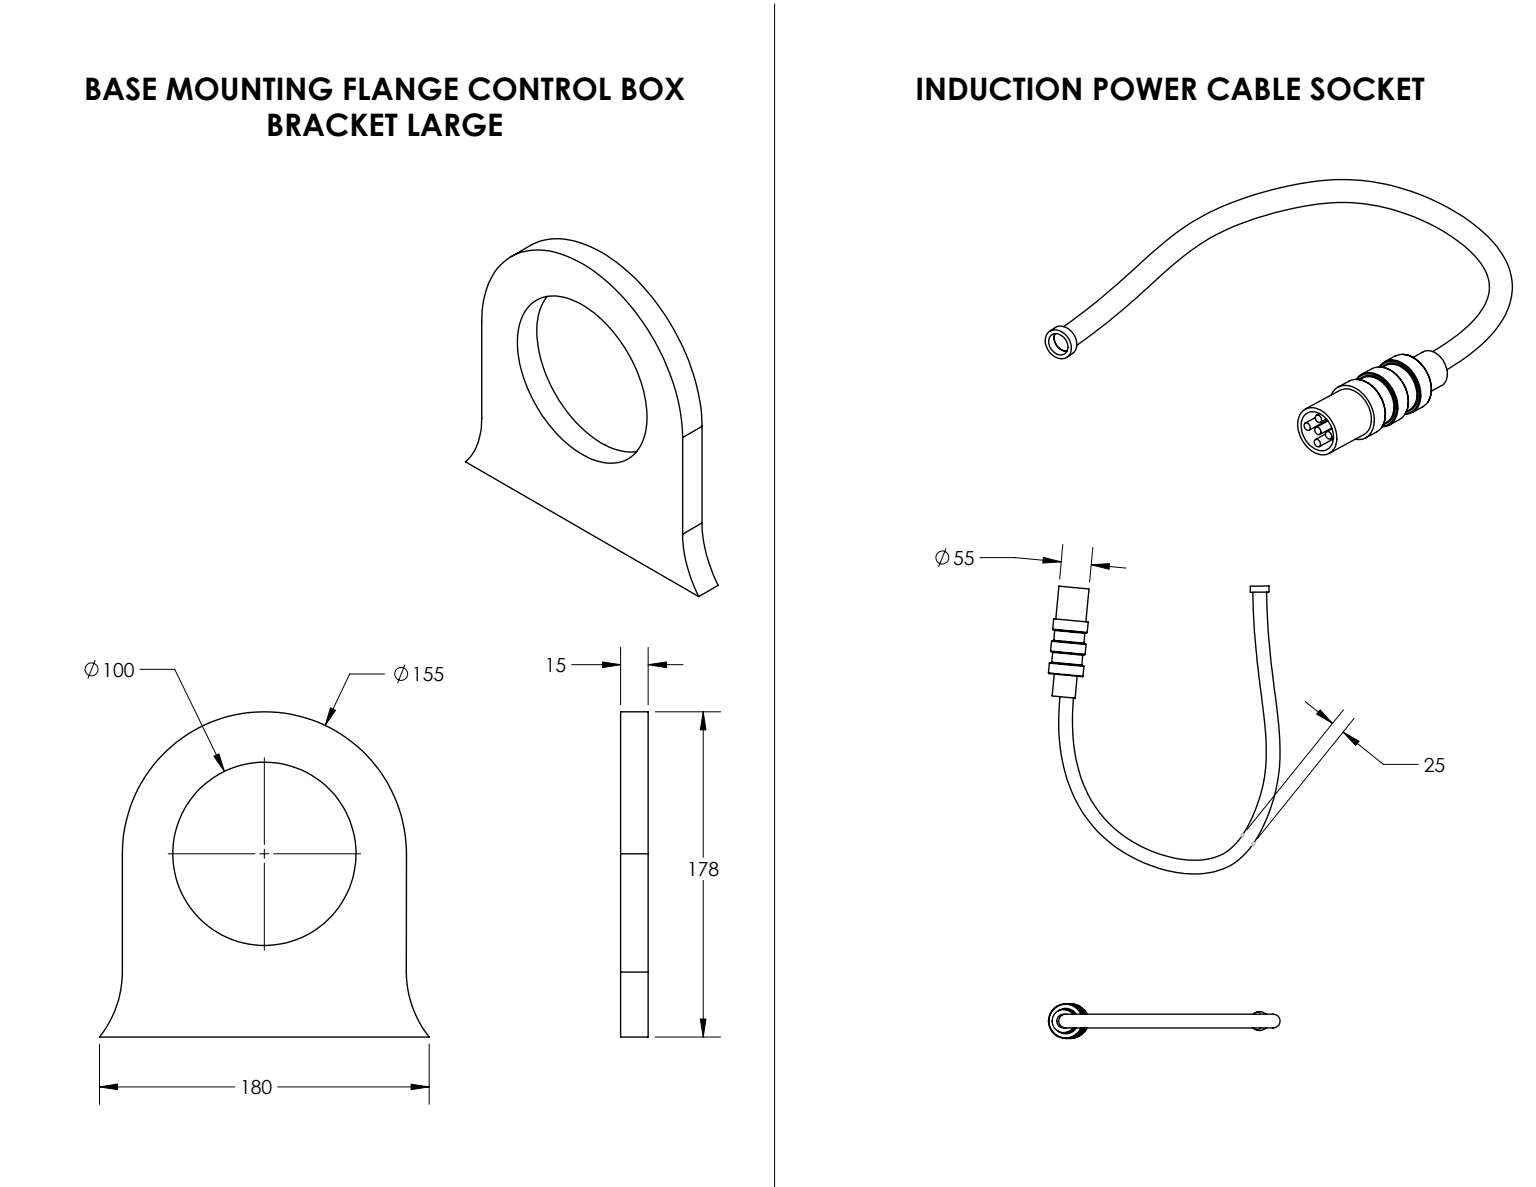
ISO-10303-21;
HEADER;
FILE_DESCRIPTION (('STEP AP214'),
    '1' );
FILE_NAME ('Induction Power Cable Socket.step',
    '2026-10-28T18:30:06',
    ( '' ),
    ( '' ),
    'SwSTEP 2.0',
    'SolidWorks 2024',
    '' );
FILE_SCHEMA (( 'AUTOMOTIVE_DESIGN' ));
ENDSEC;

DATA;
#1=CARTESIAN_POINT ( 'NONE',  ( -382.0077566144223624, 5.421010862429173848E-17, 175.3290427019271078 ) ) ;
#5=DIRECTION ( 'NONE',  ( -0.9955873536034884896, 5.465719896581968711E-31, -0.09383933793885443353 ) ) ;
#8=VERTEX_POINT ( 'NONE', #1404 ) ;
#12=DIRECTION ( 'NONE',  ( -0.09383933793885568253, 2.673190762809473730E-31, 0.9955873536034882676 ) ) ;
#17=CARTESIAN_POINT ( 'NONE',  ( -86.97194166595129161, 3.740497495074990297E-15, 531.0655262460708173 ) ) ;
#18=CARTESIAN_POINT ( 'NONE',  ( -367.0460729392618759, 0.000000000000000000, 268.0688838304710089 ) ) ;
#19=AXIS2_PLACEMENT_3D ( 'NONE', #2675, #4355, #3941 ) ;
#24=CIRCLE ( 'NONE', #2310, 4.382543221487789964 ) ;
#26=ORIENTED_EDGE ( 'NONE', *, *, #5308, .T. ) ;
#30=DIRECTION ( 'NONE',  ( 0.09383933793885537722, -2.626968444144180508E-31, -0.9955873536034883786 ) ) ;
#32=DIRECTION ( 'NONE',  ( 0.09383933793885537722, -2.626968444144180508E-31, -0.9955873536034883786 ) ) ;
#34=CARTESIAN_POINT ( 'NONE',  ( -346.0119820531829191, 0.000000000000000000, 118.4559012928527721 ) ) ;
#35=CIRCLE ( 'NONE', #3119, 30.50000000000124345 ) ;
#36=AXIS2_PLACEMENT_3D ( 'NONE', #3078, #3164, #1374 ) ;
#38=ORIENTED_EDGE ( 'NONE', *, *, #4267, .T. ) ;
#43=DIRECTION ( 'NONE',  ( 0.9955873536034884896, -5.462637660443545995E-31, 0.09383933793885503027 ) ) ;
#44=CARTESIAN_POINT ( 'NONE',  ( -379.2497704504713738, 6.080251870909620328E-15, 135.4117092198481487 ) ) ;
#47=EDGE_LOOP ( 'NONE', ( #4656, #3822, #3045, #5223 ) ) ;
#48=DIRECTION ( 'NONE',  ( 0.09383933793885568253, -2.673190762809473730E-31, -0.9955873536034882676 ) ) ;
#49=CARTESIAN_POINT ( 'NONE',  ( 6.585909452853061730, 3.740497495074990297E-15, 393.9228865916071527 ) ) ;
#55=FACE_BOUND ( 'NONE', #4165, .T. ) ;
#60=ADVANCED_FACE ( 'NONE', ( #4394, #2277 ), #4750, .F. ) ;
#63=CARTESIAN_POINT ( 'NONE',  ( 11.81831109762766729, -25.00000000000000355, 46.95220429669349471 ) ) ;
#70=DIRECTION ( 'NONE',  ( 0.09383933793885537722, -2.626968444144180508E-31, -0.9955873536034883786 ) ) ;
#71=CARTESIAN_POINT ( 'NONE',  ( -13.34676807733242754, 3.807633061153780218E-15, 36.33529372355719289 ) ) ;
#75=CARTESIAN_POINT ( 'NONE',  ( -299.8611223228758149, 3.740497495074990297E-15, 439.6443911606511392 ) ) ;
#76=CARTESIAN_POINT ( 'NONE',  ( -80.59222536594943165, -24.99999999999981881, 529.1597157429057461 ) ) ;
#78=EDGE_CURVE ( 'NONE', #3915, #4669, #546, .T. ) ;
#80=ORIENTED_EDGE ( 'NONE', *, *, #160, .F. ) ;
#81=LINE ( 'NONE', #5048, #3867 ) ;
#82=ORIENTED_EDGE ( 'NONE', *, *, #2341, .F. ) ;
#83=CARTESIAN_POINT ( 'NONE',  ( -30.63277980166695258, 0.000000000000000000, 527.1358351633697339 ) ) ;
#84=ORIENTED_EDGE ( 'NONE', *, *, #1033, .T. ) ;
#85=EDGE_CURVE ( 'NONE', #3013, #195, #2089, .T. ) ;
#87=CARTESIAN_POINT ( 'NONE',  ( -198.3455225866221667, -25.00000000000003197, 518.3576047634796851 ) ) ;
#88=CARTESIAN_POINT ( 'NONE',  ( -72.60637664584184847, 3.252606517456513302E-16, 552.9197695054128872 ) ) ;
#91=EDGE_LOOP ( 'NONE', ( #1303, #4558, #3690, #426 ) ) ;
#92=ORIENTED_EDGE ( 'NONE', *, *, #2910, .T. ) ;
#94=CARTESIAN_POINT ( 'NONE',  ( -328.0684036055322963, 2.759321206427281912E-15, 40.79703369235946298 ) ) ;
#95=FACE_OUTER_BOUND ( 'NONE', #4381, .T. ) ;
#97=CYLINDRICAL_SURFACE ( 'NONE', #5382, 27.43532828739476415 ) ;
#98=ORIENTED_EDGE ( 'NONE', *, *, #2578, .T. ) ;
#100=CARTESIAN_POINT ( 'NONE',  ( -16.96312831416361533, -24.99999999999981881, 463.2830513152442222 ) ) ;
#101=DIRECTION ( 'NONE',  ( 0.09383933793885568253, -2.673190762809473730E-31, -0.9955873536034882676 ) ) ;
#102=AXIS2_PLACEMENT_3D ( 'NONE', #3097, #2631, #4309 ) ;
#104=AXIS2_PLACEMENT_3D ( 'NONE', #682, #917, #4326 ) ;
#110=CARTESIAN_POINT ( 'NONE',  ( -285.5643670724598451, 2.222614453595284090E-15, 494.2304181244439292 ) ) ;
#111=EDGE_CURVE ( 'NONE', #1596, #1814, #592, .T. ) ;
#113=CARTESIAN_POINT ( 'NONE',  ( -336.1069982926118769, 1.517883041479706208E-15, 349.6877309229317916 ) ) ;
#114=AXIS2_PLACEMENT_3D ( 'NONE', #1904, #666, #4466 ) ;
#115=CARTESIAN_POINT ( 'NONE',  ( -364.1439395362590972, 2.398458366376004494E-13, 237.2787335496881553 ) ) ;
#117=CIRCLE ( 'NONE', #1187, 31.50000000000125766 ) ;
#119=ORIENTED_EDGE ( 'NONE', *, *, #3733, .F. ) ;
#120=ORIENTED_EDGE ( 'NONE', *, *, #4299, .T. ) ;
#121=DIRECTION ( 'NONE',  ( 0.9998833722232041143, -6.898681060795032408E-31, -0.01527226085271977431 ) ) ;
#124=MECHANICAL_DESIGN_GEOMETRIC_PRESENTATION_REPRESENTATION('',(#1085),#3988);
#129=EDGE_CURVE ( 'NONE', #2973, #1648, #4118, .T. ) ;
#130=EDGE_CURVE ( 'NONE', #8, #1142, #2447, .T. ) ;
#134=CARTESIAN_POINT ( 'NONE',  ( 23.50217280487988347, -24.99999999999981881, 428.9062724124379997 ) ) ;
#136=DIRECTION ( 'NONE',  ( -0.09383933793885536334, 2.611561004589082183E-31, 0.9955873536034882676 ) ) ;
#137=CARTESIAN_POINT ( 'NONE',  ( -49.96441683051505578, 2.222614453595284090E-15, 542.4422122871075089 ) ) ;
#139=ORIENTED_EDGE ( 'NONE', *, *, #3662, .F. ) ;
#140=CARTESIAN_POINT ( 'NONE',  ( -334.2906958041416488, 0.000000000000000000, 430.9840019716568804 ) ) ;
#144=CIRCLE ( 'NONE', #4108, 28.50000000000127898 ) ;
#149=CARTESIAN_POINT ( 'NONE',  ( -0.8482259245422840710, 2.276824562219559311E-15, 36.14439046289818691 ) ) ;
#151=( NAMED_UNIT ( * ) PLANE_ANGLE_UNIT ( ) SI_UNIT ( $, .RADIAN. ) );
#155=DIRECTION ( 'NONE',  ( 0.01527226085271972227, 2.095411779493299033E-31, 0.9998833722232041143 ) ) ;
#156=EDGE_CURVE ( 'NONE', #4669, #533, #2181, .T. ) ;
#157=CARTESIAN_POINT ( 'NONE',  ( -57.28677601057306390, -24.99999999999981881, 546.4981013186294376 ) ) ;
#158=CARTESIAN_POINT ( 'NONE',  ( -314.5571410767332736, 5.421010862426289575E-17, 120.4162530843239978 ) ) ;
#160=EDGE_CURVE ( 'NONE', #4568, #5281, #4983, .T. ) ;
#161=ADVANCED_FACE ( 'NONE', ( #1208 ), #3224, .T. ) ;
#162=EDGE_LOOP ( 'NONE', ( #316, #3364, #1642, #4137 ) ) ;
#163=AXIS2_PLACEMENT_3D ( 'NONE', #847, #4231, #4697 ) ;
#164=CARTESIAN_POINT ( 'NONE',  ( -364.1439395362591540, 2.222614453595284090E-15, 237.2787335496894343 ) ) ;
#166=EDGE_CURVE ( 'NONE', #533, #4705, #424, .T. ) ;
#168=CARTESIAN_POINT ( 'NONE',  ( -207.8397519515728504, 5.421010862427522170E-17, 541.5412455041541762 ) ) ;
#169=EDGE_LOOP ( 'NONE', ( #2313, #1592, #1135, #4605 ) ) ;
#171=DIRECTION ( 'NONE',  ( -0.9955873536034882676, 5.273458392682099492E-31, -0.09383933793885600172 ) ) ;
#173=ORIENTED_EDGE ( 'NONE', *, *, #2818, .F. ) ;
#174=FACE_BOUND ( 'NONE', #3528, .T. ) ;
#176=DIRECTION ( 'NONE',  ( -0.09383933793885568253, 2.673190762809473730E-31, 0.9955873536034882676 ) ) ;
#178=AXIS2_PLACEMENT_3D ( 'NONE', #5393, #3795, #1600 ) ;
#181=CARTESIAN_POINT ( 'NONE',  ( 18.31346110193259946, -24.99999999999981881, 444.2932575970297648 ) ) ;
#183=ADVANCED_FACE ( 'NONE', ( #2387 ), #4883, .T. ) ;
#186=CARTESIAN_POINT ( 'NONE',  ( 29.77542608467487995, 25.00000000000000355, 249.2409987768023711 ) ) ;
#189=CARTESIAN_POINT ( 'NONE',  ( 34.60640066538617532, 25.00000000000018474, 295.6817845355782879 ) ) ;
#190=ORIENTED_EDGE ( 'NONE', *, *, #2199, .F. ) ;
#193=DIRECTION ( 'NONE',  ( -0.09383933793885568253, 2.673190762809473730E-31, 0.9955873536034882676 ) ) ;
#194=AXIS2_PLACEMENT_3D ( 'NONE', #2516, #803, #5003 ) ;
#195=VERTEX_POINT ( 'NONE', #2772 ) ;
#196=VECTOR ( 'NONE', #4824, 1000.000000000000000 ) ;
#198=ORIENTED_EDGE ( 'NONE', *, *, #4878, .F. ) ;
#199=DIRECTION ( 'NONE',  ( 0.09383933793885537722, -2.626968444144180508E-31, -0.9955873536034883786 ) ) ;
#205=CYLINDRICAL_SURFACE ( 'NONE', #5207, 31.50000000000125766 ) ;
#209=CIRCLE ( 'NONE', #1527, 1.000000000000000888 ) ;
#210=CARTESIAN_POINT ( 'NONE',  ( 12.58979647763662513, -25.00000000000000355, 97.46177917735926144 ) ) ;
#214=AXIS2_PLACEMENT_3D ( 'NONE', #4438, #1050, #3151 ) ;
#216=CARTESIAN_POINT ( 'NONE',  ( -36.58361131987991399, 0.000000000000000000, 532.6725316595221784 ) ) ;
#218=CARTESIAN_POINT ( 'NONE',  ( 24.85474708473260108, -25.00000000000000355, 216.1905617304888665 ) ) ;
#222=CARTESIAN_POINT ( 'NONE',  ( 10.82492224058160879, 25.00000000000018474, 312.2165827548579387 ) ) ;
#223=ORIENTED_EDGE ( 'NONE', *, *, #2066, .T. ) ;
#224=EDGE_CURVE ( 'NONE', #3599, #1199, #1643, .T. ) ;
#229=VERTEX_POINT ( 'NONE', #3605 ) ;
#236=CARTESIAN_POINT ( 'NONE',  ( -371.4494611792977139, 5.636683259291083957E-15, 95.96964117815871020 ) ) ;
#237=FACE_OUTER_BOUND ( 'NONE', #3374, .T. ) ;
#240=CARTESIAN_POINT ( 'NONE',  ( -330.1866567701607096, -25.00000000000003197, 374.2973685668110306 ) ) ;
#245=CARTESIAN_POINT ( 'NONE',  ( 33.59898979596707136, 25.00000000000018474, 384.0431050523492900 ) ) ;
#247=CARTESIAN_POINT ( 'NONE',  ( 8.821273309634928950, -24.99999999999981881, 380.5076279642381110 ) ) ;
#248=CARTESIAN_POINT ( 'NONE',  ( 11.81831109762784315, 2.222614453595197709E-15, 46.95220429669362261 ) ) ;
#249=VERTEX_POINT ( 'NONE', #355 ) ;
#250=CARTESIAN_POINT ( 'NONE',  ( -52.92425795465503313, 25.00000000000018474, 513.6488213284155790 ) ) ;
#251=VERTEX_POINT ( 'NONE', #3663 ) ;
#253=CARTESIAN_POINT ( 'NONE',  ( -344.9797493358557858, 2.222614453595284090E-15, 107.5044404032143888 ) ) ;
#255=ADVANCED_FACE ( 'NONE', ( #1536 ), #3514, .F. ) ;
#257=ORIENTED_EDGE ( 'NONE', *, *, #966, .F. ) ;
#262=DIRECTION ( 'NONE',  ( -0.09383933793885568253, 2.673190762809473730E-31, 0.9955873536034882676 ) ) ;
#264=CYLINDRICAL_SURFACE ( 'NONE', #2932, 27.50000000000126121 ) ;
#268=DIRECTION ( 'NONE',  ( 0.09383933793885568253, -2.673190762809473730E-31, -0.9955873536034882676 ) ) ;
#271=CARTESIAN_POINT ( 'NONE',  ( -122.4270646331732451, 25.00000000000018474, 560.5113017241552598 ) ) ;
#273=CARTESIAN_POINT ( 'NONE',  ( -360.7307227603797060, -24.99999999999981881, 354.4373729494859049 ) ) ;
#274=CARTESIAN_POINT ( 'NONE',  ( -49.96441683051505578, 2.222614453595284090E-15, 542.4422122871075089 ) ) ;
#275=EDGE_CURVE ( 'NONE', #3236, #249, #1125, .T. ) ;
#276=VERTEX_POINT ( 'NONE', #5095 ) ;
#277=CARTESIAN_POINT ( 'NONE',  ( -207.8397519515722252, 24.99999999999997158, 541.5412455041529256 ) ) ;
#278=VERTEX_POINT ( 'NONE', #899 ) ;
#279=CARTESIAN_POINT ( 'NONE',  ( -383.0971833059647338, 3.911847525938617771E-15, 176.2307907175917308 ) ) ;
#280=CARTESIAN_POINT ( 'NONE',  ( 11.81831109762784315, 2.222614453595197709E-15, 46.95220429669362261 ) ) ;
#281=VERTEX_POINT ( 'NONE', #1660 ) ;
#283=EDGE_LOOP ( 'NONE', ( #1020, #3448, #92, #3790 ) ) ;
#288=CARTESIAN_POINT ( 'NONE',  ( -316.8209294095171913, 2.276824562219560495E-15, 101.1186672634072750 ) ) ;
#291=AXIS2_PLACEMENT_3D ( 'NONE', #883, #526, #2643 ) ;
#294=CYLINDRICAL_SURFACE ( 'NONE', #2881, 31.50000000000125766 ) ;
#302=AXIS2_PLACEMENT_3D ( 'NONE', #761, #354, #430 ) ;
#304=CARTESIAN_POINT ( 'NONE',  ( -16.96312831416361533, 25.00000000000018474, 463.2830513152442222 ) ) ;
#305=CARTESIAN_POINT ( 'NONE',  ( -174.3534642324312358, -24.99999999999981881, 552.7876087698487027 ) ) ;
#306=DIRECTION ( 'NONE',  ( -0.09383933793885536334, 2.626968444144180070E-31, 0.9955873536034882676 ) ) ;
#310=CARTESIAN_POINT ( 'NONE',  ( 10.82492224058167984, 3.740497495074990297E-15, 312.2165827548582229 ) ) ;
#313=DIRECTION ( 'NONE',  ( -0.09383933793885536334, 2.626968444144180070E-31, 0.9955873536034882676 ) ) ;
#316=ORIENTED_EDGE ( 'NONE', *, *, #4299, .F. ) ;
#318=DIRECTION ( 'NONE',  ( 0.09383933793885568253, -2.673190762809473730E-31, -0.9955873536034882676 ) ) ;
#319=DIRECTION ( 'NONE',  ( -0.9955873536034883786, 5.430490990731020552E-31, -0.09383933793885548824 ) ) ;
#320=EDGE_CURVE ( 'NONE', #4212, #3680, #2499, .T. ) ;
#321=DIRECTION ( 'NONE',  ( -0.09383933793885537722, 2.626968444144180508E-31, 0.9955873536034883786 ) ) ;
#322=CARTESIAN_POINT ( 'NONE',  ( -353.4921497144319460, 2.222614453595284090E-15, 38.40071206960160310 ) ) ;
#324=CARTESIAN_POINT ( 'NONE',  ( -0.6802310551622114954, 2.222614453595284090E-15, 47.14310755735262859 ) ) ;
#325=DIRECTION ( 'NONE',  ( 0.09383933793885568253, -2.673190762809473730E-31, -0.9955873536034882676 ) ) ;
#326=CARTESIAN_POINT ( 'NONE',  ( -285.5643670724598451, 2.222614453595284090E-15, 494.2304181244439292 ) ) ;
#327=DIRECTION ( 'NONE',  ( -0.9998833722232041143, 6.892903270961872452E-31, 0.01527226085271972227 ) ) ;
#328=CIRCLE ( 'NONE', #4621, 12.50000000000009237 ) ;
#330=EDGE_CURVE ( 'NONE', #4669, #1438, #1570, .T. ) ;
#331=DIRECTION ( 'NONE',  ( 0.09383933793885568253, -2.673190762809473730E-31, -0.9955873536034882676 ) ) ;
#332=CARTESIAN_POINT ( 'NONE',  ( -339.2542556961734590, 25.00000000000018474, 239.6247169981589309 ) ) ;
#333=CARTESIAN_POINT ( 'NONE',  ( 31.14585677005056041, -24.99999999999981881, 398.7793066466517757 ) ) ;
#335=EDGE_CURVE ( 'NONE', #2651, #3875, #4642, .T. ) ;
#336=TOROIDAL_SURFACE ( 'NONE', #766, 23.00000000000115108, 2.000000000000000000 ) ;
#338=CARTESIAN_POINT ( 'NONE',  ( 6.585909452840001954, 25.00000000000018474, 393.9228865916072664 ) ) ;
#341=CARTESIAN_POINT ( 'NONE',  ( -363.6733932745749485, 2.759321206427299267E-15, 99.71587303862519036 ) ) ;
#342=VERTEX_POINT ( 'NONE', #3413 ) ;
#343=ORIENTED_EDGE ( 'NONE', *, *, #1465, .T. ) ;
#344=DIRECTION ( 'NONE',  ( -0.9955873536034882676, 5.484003909441392533E-31, -0.09383933793885569641 ) ) ;
#346=DIRECTION ( 'NONE',  ( -0.9955873536034884896, 5.273458392682100368E-31, -0.09383933793885443353 ) ) ;
#349=ORIENTED_EDGE ( 'NONE', *, *, #728, .T. ) ;
#350=ORIENTED_EDGE ( 'NONE', *, *, #320, .T. ) ;
#353=CARTESIAN_POINT ( 'NONE',  ( 16.14979140325228357, 2.276824562219547873E-15, 35.88476202840195839 ) ) ;
#354=DIRECTION ( 'NONE',  ( 0.09383933793885568253, -2.673190762809473730E-31, -0.9955873536034882676 ) ) ;
#355=CARTESIAN_POINT ( 'NONE',  ( -334.2354697480813002, 2.276824562219556945E-15, 40.21575531256979019 ) ) ;
#356=CARTESIAN_POINT ( 'NONE',  ( -364.1439395362590403, 25.00000000000018474, 237.2787335496889227 ) ) ;
#358=CARTESIAN_POINT ( 'NONE',  ( -354.3266237013149862, 5.421010862427522170E-17, 381.2801272015580025 ) ) ;
#360=CARTESIAN_POINT ( 'NONE',  ( -52.92425795464261995, 3.794707603699265519E-15, 513.6488213284153517 ) ) ;
#361=ORIENTED_EDGE ( 'NONE', *, *, #2818, .T. ) ;
#362=DIRECTION ( 'NONE',  ( 0.01527226085271977431, 2.087708059715749652E-31, 0.9998833722232041143 ) ) ;
#365=EDGE_CURVE ( 'NONE', #1937, #3674, #2269, .T. ) ;
#366=ORIENTED_EDGE ( 'NONE', *, *, #1513, .F. ) ;
#370=CARTESIAN_POINT ( 'NONE',  ( -374.3862216308840516, 1.527175779051622645E-29, 115.7814801615950984 ) ) ;
#371=ORIENTED_EDGE ( 'NONE', *, *, #3784, .F. ) ;
#374=CARTESIAN_POINT ( 'NONE',  ( -344.1351952944061168, 5.421010862427522170E-17, 98.54415422078321285 ) ) ;
#376=LINE ( 'NONE', #452, #4092 ) ;
#378=CIRCLE ( 'NONE', #1955, 2.000000000000001776 ) ;
#379=FACE_OUTER_BOUND ( 'NONE', #2146, .T. ) ;
#381=CARTESIAN_POINT ( 'NONE',  ( -8.629236981521737349, 1.572093150103981429E-15, 142.6115645898827893 ) ) ;
#383=CARTESIAN_POINT ( 'NONE',  ( -80.60298687151718866, 25.00000000000018474, 555.2885198911441194 ) ) ;
#384=CARTESIAN_POINT ( 'NONE',  ( -30.63277980166695258, 0.000000000000000000, 527.1358351633697339 ) ) ;
#385=CIRCLE ( 'NONE', #731, 1.000000000000000888 ) ;
#390=AXIS2_PLACEMENT_3D ( 'NONE', #820, #4287, #2907 ) ;
#391=DIRECTION ( 'NONE',  ( -0.09383933793885537722, 2.626968444144180508E-31, 0.9955873536034883786 ) ) ;
#394=CIRCLE ( 'NONE', #2942, 22.67218956682437536 ) ;
#397=DIRECTION ( 'NONE',  ( -0.9955873536034882676, 0.000000000000000000, -0.09383933793885600172 ) ) ;
#398=DIRECTION ( 'NONE',  ( -1.000000000000000000, -1.219242865862094703E-16, 0.000000000000000000 ) ) ;
#399=EDGE_CURVE ( 'NONE', #1903, #2695, #1029, .T. ) ;
#401=CARTESIAN_POINT ( 'NONE',  ( -344.1351952944061168, 5.421010862427522170E-17, 98.54415422078321285 ) ) ;
#402=ADVANCED_FACE ( 'NONE', ( #4799 ), #2223, .F. ) ;
#403=ADVANCED_FACE ( 'NONE', ( #5233 ), #4724, .T. ) ;
#409=DIRECTION ( 'NONE',  ( 0.09383933793885568253, -2.673190762809473730E-31, -0.9955873536034882676 ) ) ;
#410=CARTESIAN_POINT ( 'NONE',  ( -312.0566616799237067, 1.517883041479706208E-15, 419.2731246273846182 ) ) ;
#411=CARTESIAN_POINT ( 'NONE',  ( -52.92425795464261995, 3.794707603699265519E-15, 513.6488213284153517 ) ) ;
#415=CARTESIAN_POINT ( 'NONE',  ( -383.0033439680259448, 3.911847525938617771E-15, 175.2352033639882620 ) ) ;
#416=CARTESIAN_POINT ( 'NONE',  ( -334.2354697480813002, -14.95948628165117178, 40.21575531256979019 ) ) ;
#420=CARTESIAN_POINT ( 'NONE',  ( -316.6216065113882223, 2.222614453595267129E-15, 142.3191748636001250 ) ) ;
#424=CIRCLE ( 'NONE', #1120, 28.50000000000127542 ) ;
#425=EDGE_LOOP ( 'NONE', ( #1381, #3302, #84, #3412 ) ) ;
#426=ORIENTED_EDGE ( 'NONE', *, *, #330, .T. ) ;
#429=DIRECTION ( 'NONE',  ( 0.09383933793885568253, -2.673190762809473730E-31, -0.9955873536034882676 ) ) ;
#430=DIRECTION ( 'NONE',  ( -0.9955873536034884896, 0.000000000000000000, -0.09383933793885443353 ) ) ;
#431=CIRCLE ( 'NONE', #178, 4.382543221487789964 ) ;
#432=CARTESIAN_POINT ( 'NONE',  ( -5.157059352426552223, 3.740497495074990297E-15, 435.5986320196309975 ) ) ;
#433=CARTESIAN_POINT ( 'NONE',  ( -52.92425795463013571, -24.99999999999981881, 513.6488213284161475 ) ) ;
#436=ORIENTED_EDGE ( 'NONE', *, *, #4267, .F. ) ;
#437=DIRECTION ( 'NONE',  ( 1.000000000000000000, -3.851859888774468203E-31, 0.000000000000000000 ) ) ;
#445=PLANE ( 'NONE',  #3284 ) ;
#446=DIRECTION ( 'NONE',  ( -0.09383933793885537722, 2.626968444144180508E-31, 0.9955873536034883786 ) ) ;
#448=ORIENTED_EDGE ( 'NONE', *, *, #1946, .T. ) ;
#452=CARTESIAN_POINT ( 'NONE',  ( -373.3906342772800713, 3.367778697655401562E-15, 115.8753194995341289 ) ) ;
#454=ORIENTED_EDGE ( 'NONE', *, *, #5175, .F. ) ;
#457=CARTESIAN_POINT ( 'NONE',  ( -268.5984117390373171, -25.00000000000003197, 475.6392848759601293 ) ) ;
#459=CIRCLE ( 'NONE', #5192, 31.50000000000125766 ) ;
#462=EDGE_CURVE ( 'NONE', #1438, #4705, #1389, .T. ) ;
#463=VERTEX_POINT ( 'NONE', #4747 ) ;
#464=VECTOR ( 'NONE', #4868, 1000.000000000000114 ) ;
#469=CARTESIAN_POINT ( 'NONE',  ( -347.8887688119603467, 2.222614453595284090E-15, 138.3676483649222178 ) ) ;
#470=AXIS2_PLACEMENT_3D ( 'NONE', #2096, #4628, #2978 ) ;
#472=ORIENTED_EDGE ( 'NONE', *, *, #2175, .T. ) ;
#475=CIRCLE ( 'NONE', #1688, 30.50000000000113332 ) ;
#476=AXIS2_PLACEMENT_3D ( 'NONE', #322, #4926, #4094 ) ;
#477=DIRECTION ( 'NONE',  ( 0.09383933793885568253, -2.673190762809473730E-31, -0.9955873536034882676 ) ) ;
#478=CARTESIAN_POINT ( 'NONE',  ( -330.1866567701607096, -25.00000000000003197, 374.2973685668110306 ) ) ;
#480=DIRECTION ( 'NONE',  ( -0.9955873536034882676, 5.498529991225538217E-31, -0.09383933793885536334 ) ) ;
#481=CIRCLE ( 'NONE', #740, 30.50000000000124345 ) ;
#485=ADVANCED_FACE ( 'NONE', ( #3976 ), #336, .T. ) ;
#487=CARTESIAN_POINT ( 'NONE',  ( -351.6423423295148041, 5.421010862427522170E-17, 178.1911425090623311 ) ) ;
#488=CIRCLE ( 'NONE', #4525, 12.50000000000003197 ) ;
#489=FACE_OUTER_BOUND ( 'NONE', #91, .T. ) ;
#493=CARTESIAN_POINT ( 'NONE',  ( -107.0991749147294172, 1.572093150103981429E-15, 535.0680222229615310 ) ) ;
#494=CARTESIAN_POINT ( 'NONE',  ( -39.32426838447570816, -24.99999999999981881, 499.4571537926179872 ) ) ;
#497=EDGE_LOOP ( 'NONE', ( #1461, #2820 ) ) ;
#501=CARTESIAN_POINT ( 'NONE',  ( 35.78913469918393275, 25.00000000000018474, 310.6402212931347435 ) ) ;
#503=CARTESIAN_POINT ( 'NONE',  ( -152.2642418386349163, 3.740497495074990297E-15, 532.1805559224781064 ) ) ;
#504=CARTESIAN_POINT ( 'NONE',  ( -207.8397519515728504, 5.421010862427522170E-17, 541.5412455041541762 ) ) ;
#506=TOROIDAL_SURFACE ( 'NONE', #1909, 30.50000000000110845, 1.000000000000000000 ) ;
#507=ORIENTED_EDGE ( 'NONE', *, *, #2250, .T. ) ;
#511=DIRECTION ( 'NONE',  ( -0.9955873536034884896, 5.452307672560235798E-31, -0.09383933793885443353 ) ) ;
#513=DIRECTION ( 'NONE',  ( -0.09383933793885568253, 2.673190762809473730E-31, 0.9955873536034882676 ) ) ;
#514=DIRECTION ( 'NONE',  ( -0.09383933793885537722, 2.626968444144180508E-31, 0.9955873536034883786 ) ) ;
#516=CARTESIAN_POINT ( 'NONE',  ( -0.8482259245422840710, 2.276824562219559311E-15, 36.14439046289818691 ) ) ;
#517=CARTESIAN_POINT ( 'NONE',  ( -80.59222536594906217, 3.740497495074990297E-15, 529.1597157429033587 ) ) ;
#521=DIRECTION ( 'NONE',  ( -0.09383933793885536334, 2.611561004589082183E-31, 0.9955873536034882676 ) ) ;
#523=ORIENTED_EDGE ( 'NONE', *, *, #365, .T. ) ;
#524=CARTESIAN_POINT ( 'NONE',  ( 33.59898979596731294, 5.421010862427522170E-17, 384.0431050523496310 ) ) ;
#525=EDGE_LOOP ( 'NONE', ( #1580, #4189, #4442, #82 ) ) ;
#526=DIRECTION ( 'NONE',  ( 0.09383933793885568253, -2.673190762809473730E-31, -0.9955873536034882676 ) ) ;
#527=CARTESIAN_POINT ( 'NONE',  ( -342.0170653153610374, -24.99999999999981881, 268.9367132353194734 ) ) ;
#528=CARTESIAN_POINT ( 'NONE',  ( -360.7307227603793649, 2.222614453595284090E-15, 354.4373729494858480 ) ) ;
#533=VERTEX_POINT ( 'NONE', #4725 ) ;
#535=DIRECTION ( 'NONE',  ( -0.09383933793885568253, 2.673190762809473730E-31, 0.9955873536034882676 ) ) ;
#536=DIRECTION ( 'NONE',  ( -0.9955873536034884896, 5.462637660443545995E-31, -0.09383933793885503027 ) ) ;
#537=DIRECTION ( 'NONE',  ( 0.09383933793885537722, -2.626968444144180508E-31, -0.9955873536034883786 ) ) ;
#538=FACE_BOUND ( 'NONE', #4829, .T. ) ;
#539=ORIENTED_EDGE ( 'NONE', *, *, #2452, .T. ) ;
#540=ADVANCED_FACE ( 'NONE', ( #3272 ), #4444, .T. ) ;
#541=DIRECTION ( 'NONE',  ( -0.9955873536034882676, 5.475514420260265162E-31, -0.09383933793885552987 ) ) ;
#542=CARTESIAN_POINT ( 'NONE',  ( 24.85474708473287109, 3.252606517456513302E-16, 216.1905617304896623 ) ) ;
#545=CIRCLE ( 'NONE', #2298, 27.50000000000126477 ) ;
#546=LINE ( 'NONE', #3957, #5331 ) ;
#547=CARTESIAN_POINT ( 'NONE',  ( -285.5643670724598451, 2.222614453595284090E-15, 494.2304181244439292 ) ) ;
#549=CIRCLE ( 'NONE', #4068, 31.50000000000114397 ) ;
#551=CARTESIAN_POINT ( 'NONE',  ( 18.31346110193232590, 2.222614453595284090E-15, 444.2932575970293101 ) ) ;
#553=CARTESIAN_POINT ( 'NONE',  ( -376.2630083896611382, 2.222614453595299473E-15, 135.6932272336650840 ) ) ;
#554=CARTESIAN_POINT ( 'NONE',  ( -36.58361131987991399, 0.000000000000000000, 532.6725316595221784 ) ) ;
#558=ADVANCED_FACE ( 'NONE', ( #1172 ), #294, .T. ) ;
#560=EDGE_CURVE ( 'NONE', #1398, #3650, #2785, .T. ) ;
#561=ORIENTED_EDGE ( 'NONE', *, *, #3629, .F. ) ;
#562=DIRECTION ( 'NONE',  ( 1.000000000000000000, -5.679099018122551417E-31, 0.000000000000000000 ) ) ;
#563=ADVANCED_FACE ( 'NONE', ( #4496 ), #506, .T. ) ;
#564=DIRECTION ( 'NONE',  ( 1.000000000000000000, -3.851859888774468203E-31, 0.000000000000000000 ) ) ;
#566=VECTOR ( 'NONE', #2317, 1000.000000000000000 ) ;
#570=VECTOR ( 'NONE', #12, 1000.000000000000000 ) ;
#572=CARTESIAN_POINT ( 'NONE',  ( 11.81831109762787690, 2.222614453595284090E-15, 46.95220429669389262 ) ) ;
#575=DIRECTION ( 'NONE',  ( -0.9998833722232041143, 6.779273404243020281E-31, 0.01527226085271993043 ) ) ;
#576=CARTESIAN_POINT ( 'NONE',  ( 29.77542608467492613, 2.222614453595284090E-15, 249.2409987768030533 ) ) ;
#578=CARTESIAN_POINT ( 'NONE',  ( -1.533280346156948193, 25.00000000000018474, 488.4857301958397784 ) ) ;
#581=CARTESIAN_POINT ( 'NONE',  ( 23.50217280488020677, 5.421010862427522170E-17, 428.9062724124374881 ) ) ;
#583=ORIENTED_EDGE ( 'NONE', *, *, #5188, .F. ) ;
#584=ORIENTED_EDGE ( 'NONE', *, *, #2199, .T. ) ;
#586=DIRECTION ( 'NONE',  ( -0.09383933793885568253, 2.673190762809473730E-31, 0.9955873536034882676 ) ) ;
#587=DIRECTION ( 'NONE',  ( -0.9955873536034882676, 5.406119142139367196E-31, -0.09383933793885596009 ) ) ;
#588=DIRECTION ( 'NONE',  ( 0.09383933793885537722, -2.626968444144180508E-31, -0.9955873536034883786 ) ) ;
#589=DIRECTION ( 'NONE',  ( -0.09383933793885537722, 2.611561004589082621E-31, 0.9955873536034883786 ) ) ;
#592=CIRCLE ( 'NONE', #3506, 30.50000000000113332 ) ;
#594=CARTESIAN_POINT ( 'NONE',  ( -336.1069982926114221, -24.99999999999981881, 349.6877309229307684 ) ) ;
#596=CARTESIAN_POINT ( 'NONE',  ( -338.5986743560152377, 14.95948628165116823, 39.80450035817695209 ) ) ;
#598=CARTESIAN_POINT ( 'NONE',  ( -174.3534642324304116, 5.421010862427522170E-17, 552.7876087698471110 ) ) ;
#600=ORIENTED_EDGE ( 'NONE', *, *, #966, .T. ) ;
#601=CARTESIAN_POINT ( 'NONE',  ( -80.60298687151718866, 25.00000000000018474, 555.2885198911441194 ) ) ;
#607=FACE_OUTER_BOUND ( 'NONE', #162, .T. ) ;
#612=CIRCLE ( 'NONE', #1585, 12.50000000000008704 ) ;
#613=DIRECTION ( 'NONE',  ( -0.9955873536034882676, 5.502656983963321189E-31, -0.09383933793885568253 ) ) ;
#614=CARTESIAN_POINT ( 'NONE',  ( -364.1439395362590403, -24.99999999999981881, 237.2787335496889227 ) ) ;
#615=DIRECTION ( 'NONE',  ( -1.000000000000000000, -1.219242865862094703E-16, 0.000000000000000000 ) ) ;
#616=DIRECTION ( 'NONE',  ( -0.09383933793885568253, 2.673190762809473730E-31, 0.9955873536034882676 ) ) ;
#620=DIRECTION ( 'NONE',  ( -0.09383933793885536334, 2.626968444144180070E-31, 0.9955873536034882676 ) ) ;
#622=CARTESIAN_POINT ( 'NONE',  ( -16.96312831416361533, -24.99999999999981881, 463.2830513152442222 ) ) ;
#623=ADVANCED_FACE ( 'NONE', ( #727, #3246 ), #3625, .T. ) ;
#626=CARTESIAN_POINT ( 'NONE',  ( -249.5207023207449879, 24.99999999999997158, 491.2832465756976035 ) ) ;
#629=CARTESIAN_POINT ( 'NONE',  ( -319.4206898963205958, 5.712857831165392007E-15, 140.0464821425766786 ) ) ;
#631=CIRCLE ( 'NONE', #2568, 4.382543221487789076 ) ;
#632=APPLICATION_CONTEXT ( 'automotive_design' ) ;
#633=ORIENTED_EDGE ( 'NONE', *, *, #2013, .T. ) ;
#634=AXIS2_PLACEMENT_3D ( 'NONE', #3604, #616, #3137 ) ;
#635=CIRCLE ( 'NONE', #114, 1.000000000000000888 ) ;
#636=ORIENTED_EDGE ( 'NONE', *, *, #160, .T. ) ;
#637=DIRECTION ( 'NONE',  ( -0.9955873536034882676, 5.498835694391114214E-31, -0.09383933793885514130 ) ) ;
#639=CYLINDRICAL_SURFACE ( 'NONE', #5014, 4.382543221487789964 ) ;
#640=DIRECTION ( 'NONE',  ( -0.09383933793885537722, 2.611561004589082621E-31, 0.9955873536034883786 ) ) ;
#646=CIRCLE ( 'NONE', #3297, 30.50000000000124345 ) ;
#647=DIRECTION ( 'NONE',  ( -0.09383933793885568253, 2.673190762809473730E-31, 0.9955873536034882676 ) ) ;
#648=AXIS2_PLACEMENT_3D ( 'NONE', #4556, #2819, #2024 ) ;
#649=CARTESIAN_POINT ( 'NONE',  ( -1.533280346156490337, 2.222614453595284090E-15, 488.4857301958385278 ) ) ;
#652=AXIS2_PLACEMENT_3D ( 'NONE', #2525, #3352, #4202 ) ;
#655=CARTESIAN_POINT ( 'NONE',  ( 24.85474708473260108, 25.00000000000000355, 216.1905617304888665 ) ) ;
#657=CARTESIAN_POINT ( 'NONE',  ( -68.63039925413373510, -24.99999999999981881, 524.1455590405155363 ) ) ;
#660=CARTESIAN_POINT ( 'NONE',  ( -68.63039925413373510, 25.00000000000018474, 524.1455590405155363 ) ) ;
#661=EDGE_LOOP ( 'NONE', ( #2351, #223 ) ) ;
#665=EDGE_LOOP ( 'NONE', ( #4208, #1745, #2026, #1244 ) ) ;
#666=DIRECTION ( 'NONE',  ( -1.219242865862094703E-16, 1.000000000000000000, -1.149200448409289593E-17 ) ) ;
#668=DIRECTION ( 'NONE',  ( -0.09383933793885568253, 2.673190762809473730E-31, 0.9955873536034882676 ) ) ;
#673=CARTESIAN_POINT ( 'NONE',  ( -156.9923520473269321, 0.000000000000000000, 556.8176423728721147 ) ) ;
#675=ADVANCED_FACE ( 'NONE', ( #1609 ), #834, .T. ) ;
#676=CARTESIAN_POINT ( 'NONE',  ( -340.0535087002904220, 2.276824562219573511E-15, 101.9421712359864500 ) ) ;
#677=DIRECTION ( 'NONE',  ( 0.9955873536034882676, -5.273458392682099492E-31, 0.09383933793885600172 ) ) ;
#678=CARTESIAN_POINT ( 'NONE',  ( 9.699276322990584731, 1.572093150103981429E-15, 297.8714164406039799 ) ) ;
#680=CARTESIAN_POINT ( 'NONE',  ( -156.9923520473274721, -24.99999999999981881, 556.8176423728723421 ) ) ;
#682=CARTESIAN_POINT ( 'NONE',  ( -321.3707673825458642, 3.789382846023848702E-15, 182.0488296698010231 ) ) ;
#683=ORIENTED_EDGE ( 'NONE', *, *, #3784, .T. ) ;
#684=CARTESIAN_POINT ( 'NONE',  ( -121.8424039467700055, 25.00000000000018474, 535.4314447305361000 ) ) ;
#685=EDGE_LOOP ( 'NONE', ( #5159, #4471 ) ) ;
#687=CARTESIAN_POINT ( 'NONE',  ( -0.8482259245422840710, 2.276824562219559311E-15, 36.14439046289818691 ) ) ;
#689=VERTEX_POINT ( 'NONE', #2165 ) ;
#690=CARTESIAN_POINT ( 'NONE',  ( -346.0119820531829191, 0.000000000000000000, 118.4559012928527721 ) ) ;
#693=DIRECTION ( 'NONE',  ( 0.09383933793885568253, -2.673190762809473730E-31, -0.9955873536034882676 ) ) ;
#694=CYLINDRICAL_SURFACE ( 'NONE', #1175, 27.50000000000126477 ) ;
#695=EDGE_CURVE ( 'NONE', #4705, #533, #4086, .T. ) ;
#696=CARTESIAN_POINT ( 'NONE',  ( -351.6423423295148041, 5.421010862427522170E-17, 178.1911425090623311 ) ) ;
#699=DIRECTION ( 'NONE',  ( -0.9955873536034882676, 5.452307672560243681E-31, -0.09383933793885551600 ) ) ;
#700=CARTESIAN_POINT ( 'NONE',  ( -349.1289451064980085, 2.222614453595281723E-15, 38.81196702399444121 ) ) ;
#701=CARTESIAN_POINT ( 'NONE',  ( -378.2541830968680188, 2.222614453595300261E-15, 135.5055485577871934 ) ) ;
#703=CARTESIAN_POINT ( 'NONE',  ( -360.7307227603797060, 25.00000000000018474, 354.4373729494859049 ) ) ;
#704=CARTESIAN_POINT ( 'NONE',  ( -49.96441683051505578, 2.222614453595284090E-15, 542.4422122871075089 ) ) ;
#705=CARTESIAN_POINT ( 'NONE',  ( -332.6117946626184221, -1.154691298157368797E-29, 200.0735156778482917 ) ) ;
#707=CARTESIAN_POINT ( 'NONE',  ( -8.629236981521737349, 1.572093150103981429E-15, 142.6115645898827893 ) ) ;
#709=CARTESIAN_POINT ( 'NONE',  ( -344.9797493358557858, 2.222614453595284090E-15, 107.5044404032143888 ) ) ;
#712=ORIENTED_EDGE ( 'NONE', *, *, #3398, .F. ) ;
#714=EDGE_LOOP ( 'NONE', ( #3323, #3873, #822, #4259 ) ) ;
#717=DIRECTION ( 'NONE',  ( -0.9955873536034882676, 5.502656983963321189E-31, -0.09383933793885573804 ) ) ;
#718=DIRECTION ( 'NONE',  ( -0.09383933793885568253, 2.673190762809473730E-31, 0.9955873536034882676 ) ) ;
#722=EDGE_LOOP ( 'NONE', ( #454, #1191, #2248, #349 ) ) ;
#727=FACE_BOUND ( 'NONE', #3395, .T. ) ;
#728=EDGE_CURVE ( 'NONE', #1738, #3769, #5299, .T. ) ;
#731=AXIS2_PLACEMENT_3D ( 'NONE', #1299, #4655, #1195 ) ;
#735=CIRCLE ( 'NONE', #4776, 1.000000000000000888 ) ;
#737=CARTESIAN_POINT ( 'NONE',  ( -330.1866567701607096, 24.99999999999997158, 374.2973685668110306 ) ) ;
#738=CARTESIAN_POINT ( 'NONE',  ( 12.58979647763672283, 2.222614453595284090E-15, 97.46177917736021357 ) ) ;
#740=AXIS2_PLACEMENT_3D ( 'NONE', #2001, #1202, #5261 ) ;
#741=AXIS2_PLACEMENT_3D ( 'NONE', #4332, #535, #1365 ) ;
#742=VERTEX_POINT ( 'NONE', #1225 ) ;
#743=CARTESIAN_POINT ( 'NONE',  ( -268.5984117390373171, 24.99999999999997158, 475.6392848759601293 ) ) ;
#744=VERTEX_POINT ( 'NONE', #1679 ) ;
#745=DIRECTION ( 'NONE',  ( -0.9955873536034882676, 5.498835694391114214E-31, -0.09383933793885536334 ) ) ;
#748=ORIENTED_EDGE ( 'NONE', *, *, #2583, .F. ) ;
#752=DIRECTION ( 'NONE',  ( -0.9955873536034882676, 5.498529991225532962E-31, -0.09383933793885514130 ) ) ;
#754=DIRECTION ( 'NONE',  ( -5.720779902258401340E-31, -1.000000000000000000, 2.099398147291833041E-31 ) ) ;
#756=EDGE_CURVE ( 'NONE', #1596, #3875, #4611, .T. ) ;
#757=EDGE_LOOP ( 'NONE', ( #2810, #4398 ) ) ;
#760=FACE_OUTER_BOUND ( 'NONE', #5303, .T. ) ;
#761=CARTESIAN_POINT ( 'NONE',  ( -344.4167133082243595, 14.95948628165116823, 101.5309162815936048 ) ) ;
#763=CARTESIAN_POINT ( 'NONE',  ( -105.2090356704102447, 25.00000000000018474, 560.1816718768288865 ) ) ;
#764=CARTESIAN_POINT ( 'NONE',  ( -334.2906958041416488, 0.000000000000000000, 430.9840019716568804 ) ) ;
#765=EDGE_CURVE ( 'NONE', #5037, #1126, #5401, .T. ) ;
#766=AXIS2_PLACEMENT_3D ( 'NONE', #3468, #5178, #980 ) ;
#767=EDGE_LOOP ( 'NONE', ( #3289, #3348, #3591, #1412 ) ) ;
#768=CARTESIAN_POINT ( 'NONE',  ( -35.15684241565247703, 1.843143693225357538E-15, 493.9702760599520275 ) ) ;
#769=ORIENTED_EDGE ( 'NONE', *, *, #1435, .T. ) ;
#778=CARTESIAN_POINT ( 'NONE',  ( -347.7949294740212736, 2.222614453595284090E-15, 137.3720610113191469 ) ) ;
#779=CARTESIAN_POINT ( 'NONE',  ( -351.6423423295148041, 5.421010862427522170E-17, 178.1911425090623311 ) ) ;
#781=DIRECTION ( 'NONE',  ( 0.9955873536034882676, -5.273458392682099492E-31, 0.09383933793885600172 ) ) ;
#786=DIRECTION ( 'NONE',  ( -0.09383933793885537722, 2.626968444144180508E-31, 0.9955873536034883786 ) ) ;
#789=DIRECTION ( 'NONE',  ( -0.9955873536034882676, 5.484003909441382024E-31, -0.09383933793885569641 ) ) ;
#790=CARTESIAN_POINT ( 'NONE',  ( -49.96441683051492078, 25.00000000000018474, 542.4422122871054626 ) ) ;
#791=CARTESIAN_POINT ( 'NONE',  ( 24.85474708473287109, 3.252606517456513302E-16, 216.1905617304896623 ) ) ;
#792=EDGE_CURVE ( 'NONE', #3702, #278, #5034, .T. ) ;
#798=EDGE_CURVE ( 'NONE', #1142, #3875, #3838, .T. ) ;
#799=ORIENTED_EDGE ( 'NONE', *, *, #3017, .T. ) ;
#803=DIRECTION ( 'NONE',  ( 0.09383933793885126939, -2.549931246368698080E-31, -0.9955873536034888227 ) ) ;
#807=AXIS2_PLACEMENT_3D ( 'NONE', #4815, #5198, #1443 ) ;
#809=DIRECTION ( 'NONE',  ( -0.9955873536034883786, 5.499036814894887477E-31, -0.09383933793885500252 ) ) ;
#814=CARTESIAN_POINT ( 'NONE',  ( -384.7862913888641287, 3.911847525938622504E-15, 194.1513630824538268 ) ) ;
#817=CARTESIAN_POINT ( 'NONE',  ( 9.699276322990584731, 1.572093150103981429E-15, 297.8714164406039799 ) ) ;
#818=CIRCLE ( 'NONE', #906, 12.50000000000002842 ) ;
#819=CARTESIAN_POINT ( 'NONE',  ( -48.20943979673047863, 3.740497495074990297E-15, 509.2978244404888528 ) ) ;
#820=CARTESIAN_POINT ( 'NONE',  ( -353.5191290882918338, 0.000000000000000000, 198.1028895811323025 ) ) ;
#822=ORIENTED_EDGE ( 'NONE', *, *, #399, .T. ) ;
#823=EDGE_CURVE ( 'NONE', #5244, #1903, #1884, .T. ) ;
#824=CARTESIAN_POINT ( 'NONE',  ( -344.4167133082243595, 2.222614453595284090E-15, 101.5309162815936048 ) ) ;
#826=EDGE_CURVE ( 'NONE', #3068, #742, #3306, .T. ) ;
#830=AXIS2_PLACEMENT_3D ( 'NONE', #4996, #4544, #4079 ) ;
#831=AXIS2_PLACEMENT_3D ( 'NONE', #1288, #2532, #4209 ) ;
#834=TOROIDAL_SURFACE ( 'NONE', #2937, 30.50000000000105516, 1.000000000000000000 ) ;
#836=LINE ( 'NONE', #4574, #5112 ) ;
#838=CARTESIAN_POINT ( 'NONE',  ( -0.8482259245422840710, 2.276824562219559311E-15, 36.14439046289818691 ) ) ;
#839=DIRECTION ( 'NONE',  ( 0.9955873536034882676, -5.498835694391114214E-31, 0.09383933793885514130 ) ) ;
#842=EDGE_LOOP ( 'NONE', ( #5325, #2255 ) ) ;
#847=CARTESIAN_POINT ( 'NONE',  ( -351.5485029915759583, 2.222614453595284090E-15, 177.1955551554592603 ) ) ;
#848=CARTESIAN_POINT ( 'NONE',  ( -13.17877320795229856, -25.00000000000000355, 47.33401081801169141 ) ) ;
#851=DIRECTION ( 'NONE',  ( -0.09383933793885536334, 2.611561004589082183E-31, 0.9955873536034882676 ) ) ;
#852=( LENGTH_UNIT ( ) NAMED_UNIT ( * ) SI_UNIT ( .MILLI., .METRE. ) );
#854=CIRCLE ( 'NONE', #4046, 21.00000000000012790 ) ;
#858=FACE_OUTER_BOUND ( 'NONE', #661, .T. ) ;
#859=FACE_OUTER_BOUND ( 'NONE', #4770, .T. ) ;
#860=VERTEX_POINT ( 'NONE', #4966 ) ;
#861=VERTEX_POINT ( 'NONE', #1003 ) ;
#862=ADVANCED_FACE ( 'NONE', ( #607 ), #3459, .T. ) ;
#869=EDGE_CURVE ( 'NONE', #3237, #4129, #2674, .T. ) ;
#870=CARTESIAN_POINT ( 'NONE',  ( -68.63039925413394826, 1.572093150103981429E-15, 524.1455590405157636 ) ) ;
#871=CARTESIAN_POINT ( 'NONE',  ( -107.0991749147297014, -24.99999999999981881, 535.0680222229608489 ) ) ;
#872=DIRECTION ( 'NONE',  ( 0.09383933793885568253, -2.673190762809473730E-31, -0.9955873536034882676 ) ) ;
#875=ORIENTED_EDGE ( 'NONE', *, *, #1230, .F. ) ;
#876=PLANE ( 'NONE',  #4144 ) ;
#879=ADVANCED_FACE ( 'NONE', ( #1442, #5088, #4742, #3047, #174, #3926 ), #3537, .T. ) ;
#880=ORIENTED_EDGE ( 'NONE', *, *, #965, .F. ) ;
#882=ADVANCED_FACE ( 'NONE', ( #3889 ), #3968, .F. ) ;
#883=CARTESIAN_POINT ( 'NONE',  ( -344.1351952944073105, 5.421010862427522170E-17, 98.54415422078299969 ) ) ;
#884=DIRECTION ( 'NONE',  ( 0.09383933793885126939, -2.549931246368698080E-31, -0.9955873536034888227 ) ) ;
#888=ORIENTED_EDGE ( 'NONE', *, *, #4057, .F. ) ;
#894=EDGE_CURVE ( 'NONE', #4568, #3984, #2592, .T. ) ;
#897=ADVANCED_FACE ( 'NONE', ( #1803 ), #5212, .T. ) ;
#899=CARTESIAN_POINT ( 'NONE',  ( -312.7741936558949760, 5.421010862425789758E-17, 101.5000933658572819 ) ) ;
#900=CARTESIAN_POINT ( 'NONE',  ( -8.629236981504860182, -25.00000000000000355, 142.6115645898824198 ) ) ;
#901=CARTESIAN_POINT ( 'NONE',  ( -374.2387848380886908, 2.625968386833892010E-15, 194.1410887772089779 ) ) ;
#903=AXIS2_PLACEMENT_3D ( 'NONE', #2789, #693, #346 ) ;
#906=AXIS2_PLACEMENT_3D ( 'NONE', #3293, #884, #2070 ) ;
#908=CARTESIAN_POINT ( 'NONE',  ( -344.4167133082243595, 14.95948628165116823, 101.5309162815936048 ) ) ;
#910=AXIS2_PLACEMENT_3D ( 'NONE', #5121, #513, #5150 ) ;
#911=VERTEX_POINT ( 'NONE', #2606 ) ;
#913=VECTOR ( 'NONE', #2782, 1000.000000000000114 ) ;
#915=FACE_OUTER_BOUND ( 'NONE', #3184, .T. ) ;
#916=CARTESIAN_POINT ( 'NONE',  ( 9.699276322990401766, -24.99999999999981881, 297.8714164406044915 ) ) ;
#917=DIRECTION ( 'NONE',  ( -1.219242865862094703E-16, 1.000000000000000000, -1.149200448409285278E-17 ) ) ;
#925=CARTESIAN_POINT ( 'NONE',  ( -359.3101886666408404, 0.000000000000000000, 100.1271279930180356 ) ) ;
#926=CARTESIAN_POINT ( 'NONE',  ( -380.1309698556455601, 2.222614453595300656E-15, 155.4172956298577901 ) ) ;
#929=DIRECTION ( 'NONE',  ( 0.9955873536034883786, -5.498529991225532086E-31, 0.09383933793885522456 ) ) ;
#932=CARTESIAN_POINT ( 'NONE',  ( -299.8611223228758149, 3.740497495074990297E-15, 439.6443911606511392 ) ) ;
#936=VERTEX_POINT ( 'NONE', #3096 ) ;
#938=ORIENTED_EDGE ( 'NONE', *, *, #462, .F. ) ;
#939=CARTESIAN_POINT ( 'NONE',  ( -19.78983854945498422, 2.222614453595284090E-15, 515.1268587725810448 ) ) ;
#941=CARTESIAN_POINT ( 'NONE',  ( 4.992201166475765284, -24.99999999999981881, 252.6216919286950429 ) ) ;
#942=CARTESIAN_POINT ( 'NONE',  ( -14.89480152442229688, 0.000000000000000000, 508.6517828409968729 ) ) ;
#943=DIRECTION ( 'NONE',  ( -0.9955873536034882676, 5.452307672560245432E-31, -0.09383933793885568253 ) ) ;
#946=ORIENTED_EDGE ( 'NONE', *, *, #4729, .T. ) ;
#949=CARTESIAN_POINT ( 'NONE',  ( -351.6423423295148041, 5.421010862427522170E-17, 178.1911425090623311 ) ) ;
#950=CARTESIAN_POINT ( 'NONE',  ( -377.2380471327739997, 5.590393151250686046E-15, 156.6944009972769152 ) ) ;
#951=CARTESIAN_POINT ( 'NONE',  ( -357.2727026058461206, 5.421010862427522170E-17, 237.9263837252718758 ) ) ;
#952=ORIENTED_EDGE ( 'NONE', *, *, #826, .T. ) ;
#955=CARTESIAN_POINT ( 'NONE',  ( -1.533280346156948193, -24.99999999999981881, 488.4857301958397784 ) ) ;
#957=DIRECTION ( 'NONE',  ( -0.01527226085271972227, -2.080004339938201146E-31, -0.9998833722232041143 ) ) ;
#958=DIRECTION ( 'NONE',  ( -0.9955873536034884896, 0.000000000000000000, -0.09383933793885443353 ) ) ;
#959=DIRECTION ( 'NONE',  ( 0.000000000000000000, 0.000000000000000000, 1.000000000000000000 ) ) ;
#961=EDGE_CURVE ( 'NONE', #1937, #4307, #3014, .T. ) ;
#963=CARTESIAN_POINT ( 'NONE',  ( 24.85474708473260108, 25.00000000000000355, 216.1905617304888665 ) ) ;
#965=EDGE_CURVE ( 'NONE', #3650, #1398, #1621, .T. ) ;
#966=EDGE_CURVE ( 'NONE', #2722, #2477, #2192, .T. ) ;
#967=FACE_OUTER_BOUND ( 'NONE', #1472, .T. ) ;
#968=CARTESIAN_POINT ( 'NONE',  ( -312.0566616799237067, 1.517883041479706208E-15, 419.2731246273846182 ) ) ;
#969=CARTESIAN_POINT ( 'NONE',  ( -285.5643670724598451, 2.222614453595284090E-15, 494.2304181244439292 ) ) ;
#970=CARTESIAN_POINT ( 'NONE',  ( -323.7051989975983588, 2.222614453595284090E-15, 41.20828864675230108 ) ) ;
#971=EDGE_CURVE ( 'NONE', #3674, #1937, #3559, .T. ) ;
#972=ORIENTED_EDGE ( 'NONE', *, *, #3185, .F. ) ;
#973=EDGE_LOOP ( 'NONE', ( #5370, #5420, #2966, #2980 ) ) ;
#980=DIRECTION ( 'NONE',  ( -0.9955873536034882676, 5.498529991225541720E-31, -0.09383933793885536334 ) ) ;
#981=CARTESIAN_POINT ( 'NONE',  ( 12.58979647763672283, 2.222614453595284090E-15, 97.46177917736021357 ) ) ;
#983=EDGE_CURVE ( 'NONE', #4831, #4212, #1447, .T. ) ;
#984=AXIS2_PLACEMENT_3D ( 'NONE', #2444, #5319, #699 ) ;
#987=CARTESIAN_POINT ( 'NONE',  ( -19.78983854945498422, 2.222614453595284090E-15, 515.1268587725810448 ) ) ;
#992=CARTESIAN_POINT ( 'NONE',  ( -354.3266237013149862, 5.421010862427522170E-17, 381.2801272015580025 ) ) ;
#997=CARTESIAN_POINT ( 'NONE',  ( -334.2906958041416488, 0.000000000000000000, 430.9840019716568804 ) ) ;
#998=DIRECTION ( 'NONE',  ( 0.09383933793885568253, -2.673190762809473730E-31, -0.9955873536034882676 ) ) ;
#999=AXIS2_PLACEMENT_3D ( 'NONE', #970, #1411, #171 ) ;
#1003=CARTESIAN_POINT ( 'NONE',  ( -383.8845433731994490, 1.677051647323856397E-29, 195.2407897739975624 ) ) ;
#1010=ORIENTED_EDGE ( 'NONE', *, *, #5425, .T. ) ;
#1012=AXIS2_PLACEMENT_3D ( 'NONE', #3436, #4689, #4988 ) ;
#1014=CARTESIAN_POINT ( 'NONE',  ( -36.58361131987991399, 0.000000000000000000, 532.6725316595221784 ) ) ;
#1017=CARTESIAN_POINT ( 'NONE',  ( 5.624351423727524946, 2.222614453595284090E-15, 474.0483466084679662 ) ) ;
#1018=ORIENTED_EDGE ( 'NONE', *, *, #1653, .F. ) ;
#1019=CARTESIAN_POINT ( 'NONE',  ( 23.50217280487988347, 25.00000000000018474, 428.9062724124379997 ) ) ;
#1020=ORIENTED_EDGE ( 'NONE', *, *, #1917, .F. ) ;
#1027=CARTESIAN_POINT ( 'NONE',  ( -351.5485029915759583, 2.222614453595284090E-15, 177.1955551554592603 ) ) ;
#1029=CIRCLE ( 'NONE', #2961, 1.000000000000000888 ) ;
#1030=EDGE_CURVE ( 'NONE', #1903, #5244, #3739, .T. ) ;
#1031=CARTESIAN_POINT ( 'NONE',  ( -315.9326898068451897, 4.999156891862612154E-15, 40.93645626314877717 ) ) ;
#1033=EDGE_CURVE ( 'NONE', #3599, #3314, #4433, .T. ) ;
#1034=EDGE_CURVE ( 'NONE', #3745, #744, #5128, .T. ) ;
#1035=CARTESIAN_POINT ( 'NONE',  ( -376.1691690517220081, 2.222614453595299473E-15, 134.6976398800616437 ) ) ;
#1037=CARTESIAN_POINT ( 'NONE',  ( -334.2906958041451162, -25.00000000000003197, 430.9840019716597226 ) ) ;
#1038=CARTESIAN_POINT ( 'NONE',  ( -338.5986743560152377, -14.95948628165117178, 39.80450035817695209 ) ) ;
#1039=DIRECTION ( 'NONE',  ( -0.09383933793885568253, 2.673190762809473730E-31, 0.9955873536034882676 ) ) ;
#1041=CARTESIAN_POINT ( 'NONE',  ( 31.14585677005082687, 2.222614453595284090E-15, 398.7793066466531968 ) ) ;
#1043=CARTESIAN_POINT ( 'NONE',  ( -57.28677601057306390, 25.00000000000018474, 546.4981013186294376 ) ) ;
#1048=ORIENTED_EDGE ( 'NONE', *, *, #2914, .F. ) ;
#1049=DIRECTION ( 'NONE',  ( -0.09383933793885537722, 2.626968444144180508E-31, 0.9955873536034883786 ) ) ;
#1050=DIRECTION ( 'NONE',  ( 0.01527226085271977431, 2.087708059715749652E-31, 0.9998833722232041143 ) ) ;
#1051=DIRECTION ( 'NONE',  ( 0.09383933793885537722, -2.626968444144180508E-31, -0.9955873536034883786 ) ) ;
#1052=LINE ( 'NONE', #3948, #5201 ) ;
#1053=FACE_OUTER_BOUND ( 'NONE', #2214, .T. ) ;
#1054=ORIENTED_EDGE ( 'NONE', *, *, #399, .F. ) ;
#1056=ADVANCED_FACE ( 'NONE', ( #1077 ), #5329, .T. ) ;
#1057=CARTESIAN_POINT ( 'NONE',  ( 18.31346110193232590, 2.222614453595284090E-15, 444.2932575970293101 ) ) ;
#1063=CARTESIAN_POINT ( 'NONE',  ( -367.0882437885061904, 2.222614453595284090E-15, 297.8351940652699454 ) ) ;
#1064=SHAPE_DEFINITION_REPRESENTATION ( #5391, #2334 ) ;
#1065=CARTESIAN_POINT ( 'NONE',  ( -23.53079058812344471, -24.99999999999981881, 476.4235034963351154 ) ) ;
#1067=CARTESIAN_POINT ( 'NONE',  ( -5.157059352427092236, 25.00000000000018474, 435.5986320196304860 ) ) ;
#1069=CIRCLE ( 'NONE', #3360, 31.50000000000120082 ) ;
#1073=VECTOR ( 'NONE', #5027, 1000.000000000000000 ) ;
#1074=VECTOR ( 'NONE', #2811, 1000.000000000000000 ) ;
#1075=ORIENTED_EDGE ( 'NONE', *, *, #3017, .F. ) ;
#1077=FACE_OUTER_BOUND ( 'NONE', #5137, .T. ) ;
#1079=CARTESIAN_POINT ( 'NONE',  ( -338.5986743560152377, 2.276824562219559311E-15, 39.80450035817695209 ) ) ;
#1081=CARTESIAN_POINT ( 'NONE',  ( -332.4241159867397073, 5.421010862426837463E-17, 198.0823409706411553 ) ) ;
#1082=ORIENTED_EDGE ( 'NONE', *, *, #1325, .T. ) ;
#1085=STYLED_ITEM('',(#5451),#4927);
#1089=CARTESIAN_POINT ( 'NONE',  ( -353.3314504124138011, 0.000000000000000000, 196.1117148739250808 ) ) ;
#1090=TOROIDAL_SURFACE ( 'NONE', #4175, 30.50000000000110845, 1.000000000000000000 ) ;
#1093=DIRECTION ( 'NONE',  ( -0.9955873536034883786, 5.499036814894887477E-31, -0.09383933793885500252 ) ) ;
#1094=CARTESIAN_POINT ( 'NONE',  ( 12.58979647763662513, 25.00000000000000355, 97.46177917735926144 ) ) ;
#1096=CARTESIAN_POINT ( 'NONE',  ( 23.50217280487988347, -24.99999999999981881, 428.9062724124379997 ) ) ;
#1099=CARTESIAN_POINT ( 'NONE',  ( -330.1866567701607096, 24.99999999999997158, 374.2973685668110306 ) ) ;
#1106=EDGE_LOOP ( 'NONE', ( #2899, #3300, #4791, #1762 ) ) ;
#1107=CARTESIAN_POINT ( 'NONE',  ( -17.84624325233685127, 4.358724120770097062E-15, 36.40401889739442254 ) ) ;
#1108=DIRECTION ( 'NONE',  ( 0.09383933793885568253, -2.673190762809473730E-31, -0.9955873536034882676 ) ) ;
#1109=DIRECTION ( 'NONE',  ( 0.09383933793885537722, -2.626968444144180508E-31, -0.9955873536034883786 ) ) ;
#1114=CIRCLE ( 'NONE', #4194, 17.00000000000009948 ) ;
#1119=CARTESIAN_POINT ( 'NONE',  ( -13.17877320795252238, 3.807633061153782584E-15, 47.33401081801162746 ) ) ;
#1120=AXIS2_PLACEMENT_3D ( 'NONE', #4477, #4908, #1093 ) ;
#1122=CARTESIAN_POINT ( 'NONE',  ( -268.5984117390373171, 24.99999999999997158, 475.6392848759601293 ) ) ;
#1123=CARTESIAN_POINT ( 'NONE',  ( -367.0460729392618191, -24.99999999999981881, 268.0688838304706678 ) ) ;
#1124=CARTESIAN_POINT ( 'NONE',  ( -342.9618789639491752, -14.95948628165117178, 39.39324540378412109 ) ) ;
#1125=CIRCLE ( 'NONE', #4204, 4.382543221487789964 ) ;
#1126=VERTEX_POINT ( 'NONE', #4522 ) ;
#1127=CARTESIAN_POINT ( 'NONE',  ( -342.0170653153610374, 25.00000000000018474, 268.9367132353194734 ) ) ;
#1129=ADVANCED_FACE ( 'NONE', ( #4920 ), #4814, .T. ) ;
#1130=LINE ( 'NONE', #3260, #913 ) ;
#1133=ORIENTED_EDGE ( 'NONE', *, *, #1696, .T. ) ;
#1135=ORIENTED_EDGE ( 'NONE', *, *, #826, .F. ) ;
#1139=CARTESIAN_POINT ( 'NONE',  ( -329.5232379498077080, 5.421010862427522170E-17, 102.9347045701690604 ) ) ;
#1141=DIRECTION ( 'NONE',  ( 0.09383933793885568253, -2.673190762809473730E-31, -0.9955873536034882676 ) ) ;
#1142=VERTEX_POINT ( 'NONE', #420 ) ;
#1146=CARTESIAN_POINT ( 'NONE',  ( -365.9639710083354203, 1.530808498934204340E-15, 196.9298978568966163 ) ) ;
#1148=CARTESIAN_POINT ( 'NONE',  ( -376.2299595452952303, 1.264661897981941762E-29, 193.9534101013312863 ) ) ;
#1149=CARTESIAN_POINT ( 'NONE',  ( -39.32426838450110296, 25.00000000000018474, 499.4571537926176461 ) ) ;
#1150=CARTESIAN_POINT ( 'NONE',  ( -57.28677601057280100, 3.252606517456513302E-16, 546.4981013186296650 ) ) ;
#1152=CARTESIAN_POINT ( 'NONE',  ( -13.17877320795229856, 25.00000000000000355, 47.33401081801169141 ) ) ;
#1153=ORIENTED_EDGE ( 'NONE', *, *, #5271, .T. ) ;
#1156=EDGE_CURVE ( 'NONE', #2554, #1574, #4891, .T. ) ;
#1158=ORIENTED_EDGE ( 'NONE', *, *, #2207, .T. ) ;
#1162=CYLINDRICAL_SURFACE ( 'NONE', #2574, 27.50000000000126477 ) ;
#1163=AXIS2_PLACEMENT_3D ( 'NONE', #838, #4576, #3345 ) ;
#1164=DIRECTION ( 'NONE',  ( -0.9955873536034882676, 5.475514420260265162E-31, -0.09383933793885552987 ) ) ;
#1167=CARTESIAN_POINT ( 'NONE',  ( -344.4167133082243595, 2.222614453595284090E-15, 101.5309162815936048 ) ) ;
#1168=EDGE_LOOP ( 'NONE', ( #4715, #748, #3966, #4890 ) ) ;
#1172=FACE_OUTER_BOUND ( 'NONE', #4283, .T. ) ;
#1173=FACE_OUTER_BOUND ( 'NONE', #767, .T. ) ;
#1174=DIRECTION ( 'NONE',  ( 0.9955873536034882676, -5.502656983963330823E-31, 0.09383933793885547436 ) ) ;
#1175=AXIS2_PLACEMENT_3D ( 'NONE', #34, #446, #3755 ) ;
#1179=CARTESIAN_POINT ( 'NONE',  ( -68.63039925413373510, 25.00000000000018474, 524.1455590405155363 ) ) ;
#1180=CARTESIAN_POINT ( 'NONE',  ( -223.9642223310785312, 5.421010862427522170E-17, 534.3227077389987016 ) ) ;
#1181=AXIS2_PLACEMENT_3D ( 'NONE', #2660, #2713, #2225 ) ;
#1183=AXIS2_PLACEMENT_3D ( 'NONE', #925, #4279, #511 ) ;
#1185=CARTESIAN_POINT ( 'NONE',  ( -364.1439395362590403, 25.00000000000018474, 237.2787335496889227 ) ) ;
#1187=AXIS2_PLACEMENT_3D ( 'NONE', #4006, #321, #4923 ) ;
#1188=DIRECTION ( 'NONE',  ( 0.09383933793885568253, -2.673190762809473730E-31, -0.9955873536034882676 ) ) ;
#1189=DIRECTION ( 'NONE',  ( -0.9955873536034882676, 5.498529991225543472E-31, -0.09383933793885566865 ) ) ;
#1191=ORIENTED_EDGE ( 'NONE', *, *, #2031, .F. ) ;
#1193=DIRECTION ( 'NONE',  ( -0.09383933793885568253, 2.673190762809473730E-31, 0.9955873536034882676 ) ) ;
#1195=DIRECTION ( 'NONE',  ( 1.000000000000000000, -5.720779902258384700E-31, 0.000000000000000000 ) ) ;
#1199=VERTEX_POINT ( 'NONE', #2120 ) ;
#1201=CARTESIAN_POINT ( 'NONE',  ( -264.1404626571534777, 2.222614453595284090E-15, 511.7445549721628595 ) ) ;
#1202=DIRECTION ( 'NONE',  ( 0.09383933793885537722, -2.626968444144180508E-31, -0.9955873536034883786 ) ) ;
#1203=EDGE_CURVE ( 'NONE', #860, #342, #854, .T. ) ;
#1204=ADVANCED_FACE ( 'NONE', ( #1240 ), #2364, .F. ) ;
#1206=EDGE_CURVE ( 'NONE', #278, #3702, #4220, .T. ) ;
#1207=EDGE_CURVE ( 'NONE', #2477, #3339, #1845, .T. ) ;
#1208=FACE_OUTER_BOUND ( 'NONE', #5242, .T. ) ;
#1209=CARTESIAN_POINT ( 'NONE',  ( -342.0244061588616091, 25.00000000000018474, 297.0039604601892620 ) ) ;
#1210=CARTESIAN_POINT ( 'NONE',  ( 31.14585677005082687, 2.222614453595284090E-15, 398.7793066466531968 ) ) ;
#1212=EDGE_LOOP ( 'NONE', ( #3502, #3142, #3219, #4157 ) ) ;
#1213=EDGE_LOOP ( 'NONE', ( #880, #2719 ) ) ;
#1214=CLOSED_SHELL ( 'NONE', ( #161, #183, #3754, #4160, #1928, #3466, #1769, #485, #563, #3808, #4728, #897, #1056, #1204, #2012, #3566, #1372, #4597, #4487, #3912, #3176, #3259, #5092, #4389, #2360, #4563, #3138, #1871, #5086, #60, #1765, #5253, #623, #1624, #558, #2030, #403, #4029, #5361, #675, #4962, #255, #1764, #1456, #1939, #1540, #3155, #5141, #879, #4061, #862, #2601, #540, #4760, #2106, #2608, #3346, #4967, #2180, #1129 ) ) ;
#1216=DIRECTION ( 'NONE',  ( -0.9955873536034883786, 5.498529991225534714E-31, -0.09383933793885515517 ) ) ;
#1217=EDGE_LOOP ( 'NONE', ( #1394, #3494, #4687, #1342 ) ) ;
#1221=EDGE_CURVE ( 'NONE', #4306, #742, #4913, .T. ) ;
#1225=CARTESIAN_POINT ( 'NONE',  ( -322.0642881118418472, 5.421010862426285877E-17, 200.0632413726019649 ) ) ;
#1228=EDGE_CURVE ( 'NONE', #2722, #1390, #431, .T. ) ;
#1229=CARTESIAN_POINT ( 'NONE',  ( 16.14979140325228357, 2.276824562219547873E-15, 35.88476202840195839 ) ) ;
#1230=EDGE_CURVE ( 'NONE', #463, #3842, #2802, .T. ) ;
#1231=CARTESIAN_POINT ( 'NONE',  ( 0.07030049710132768581, 1.843143693225357538E-15, 219.5055207296747710 ) ) ;
#1232=CARTESIAN_POINT ( 'NONE',  ( -299.8611223228771792, -25.00000000000003197, 439.6443911606498887 ) ) ;
#1235=LINE ( 'NONE', #3258, #3798 ) ;
#1236=CARTESIAN_POINT ( 'NONE',  ( -323.7051989975983588, 2.222614453595284090E-15, 41.20828864675230108 ) ) ;
#1238=ORIENTED_EDGE ( 'NONE', *, *, #3499, .T. ) ;
#1239=LINE ( 'NONE', #5028, #3287 ) ;
#1240=FACE_OUTER_BOUND ( 'NONE', #1378, .T. ) ;
#1241=FACE_OUTER_BOUND ( 'NONE', #3846, .T. ) ;
#1243=AXIS2_PLACEMENT_3D ( 'NONE', #4099, #4531, #2469 ) ;
#1244=ORIENTED_EDGE ( 'NONE', *, *, #2013, .F. ) ;
#1247=CARTESIAN_POINT ( 'NONE',  ( -319.3063019478910292, 4.060433389145217710E-15, 160.1459078905241427 ) ) ;
#1251=CARTESIAN_POINT ( 'NONE',  ( -63.04765821499436385, 1.843143693225357538E-15, 521.0401840782876661 ) ) ;
#1253=CARTESIAN_POINT ( 'NONE',  ( -330.1866567701584927, 3.740497495074990297E-15, 374.2973685668102917 ) ) ;
#1255=CARTESIAN_POINT ( 'NONE',  ( -5.157059352426552223, 3.740497495074990297E-15, 435.5986320196309975 ) ) ;
#1256=CARTESIAN_POINT ( 'NONE',  ( -367.0882437885061904, 2.222614453595284090E-15, 297.8351940652699454 ) ) ;
#1258=MECHANICAL_DESIGN_GEOMETRIC_PRESENTATION_REPRESENTATION('',(#1613),#4081);
#1261=CIRCLE ( 'NONE', #1695, 23.00000000000121503 ) ;
#1263=DIRECTION ( 'NONE',  ( 0.09383933793885568253, -2.673190762809473730E-31, -0.9955873536034882676 ) ) ;
#1266=EDGE_CURVE ( 'NONE', #4306, #861, #2859, .T. ) ;
#1267=AXIS2_PLACEMENT_3D ( 'NONE', #5287, #4066, #327 ) ;
#1268=PLANE ( 'NONE',  #1958 ) ;
#1270=DIRECTION ( 'NONE',  ( -0.9955873536034883786, 5.498529991225534714E-31, -0.09383933793885515517 ) ) ;
#1272=PLANE ( 'NONE',  #3800 ) ;
#1275=ORIENTED_EDGE ( 'NONE', *, *, #129, .F. ) ;
#1279=FACE_OUTER_BOUND ( 'NONE', #3860, .T. ) ;
#1280=CARTESIAN_POINT ( 'NONE',  ( -351.6423423295148041, 5.421010862427522170E-17, 178.1911425090623311 ) ) ;
#1282=CARTESIAN_POINT ( 'NONE',  ( -121.8424039465433566, -24.99999999999981881, 535.4314447305355316 ) ) ;
#1285=MANIFOLD_SOLID_BREP ( 'Boss-Extrude9', #1214 ) ;
#1288=CARTESIAN_POINT ( 'NONE',  ( -349.7655555707375470, 2.222614453595284090E-15, 158.2793954369922176 ) ) ;
#1289=( LENGTH_UNIT ( ) NAMED_UNIT ( * ) SI_UNIT ( .MILLI., .METRE. ) );
#1294=AXIS2_PLACEMENT_3D ( 'NONE', #4874, #1108, #3676 ) ;
#1296=DIRECTION ( 'NONE',  ( -0.9955873536034882676, 5.452307672560245432E-31, -0.09383933793885568253 ) ) ;
#1299=CARTESIAN_POINT ( 'NONE',  ( -383.7907040352601484, 1.677051647323856397E-29, 194.2452024203927294 ) ) ;
#1303=ORIENTED_EDGE ( 'NONE', *, *, #2452, .F. ) ;
#1304=EDGE_LOOP ( 'NONE', ( #2967, #2069, #343, #472 ) ) ;
#1305=DIRECTION ( 'NONE',  ( -0.9955873536034882676, 5.498529991225532962E-31, -0.09383933793885514130 ) ) ;
#1306=CARTESIAN_POINT ( 'NONE',  ( -353.3314504124138011, 0.000000000000000000, 196.1117148739250808 ) ) ;
#1309=FACE_OUTER_BOUND ( 'NONE', #47, .T. ) ;
#1312=CARTESIAN_POINT ( 'NONE',  ( 11.35554381053716000, 3.794707603699265519E-15, 353.5846600851142512 ) ) ;
#1315=ORIENTED_EDGE ( 'NONE', *, *, #823, .T. ) ;
#1317=AXIS2_PLACEMENT_3D ( 'NONE', #2589, #3849, #2639 ) ;
#1320=CARTESIAN_POINT ( 'NONE',  ( -382.1015959523611514, 5.421010862429199116E-17, 176.3246300555306050 ) ) ;
#1321=DIRECTION ( 'NONE',  ( -0.9955873536034882676, 5.452307672560245432E-31, -0.09383933793885568253 ) ) ;
#1322=CARTESIAN_POINT ( 'NONE',  ( -152.2642418387488874, -24.99999999999981881, 532.1805559224803801 ) ) ;
#1324=DIRECTION ( 'NONE',  ( -0.09383933793885536334, 2.611561004589082183E-31, 0.9955873536034882676 ) ) ;
#1325=EDGE_CURVE ( 'NONE', #3769, #1738, #5399, .T. ) ;
#1326=DIRECTION ( 'NONE',  ( 0.09383933793885568253, -2.673190762809473730E-31, -0.9955873536034882676 ) ) ;
#1328=EDGE_LOOP ( 'NONE', ( #3322, #1911, #2307, #683 ) ) ;
#1332=DIRECTION ( 'NONE',  ( -0.9955873536034882676, 5.498529991225538217E-31, -0.09383933793885536334 ) ) ;
#1333=FACE_OUTER_BOUND ( 'NONE', #1168, .T. ) ;
#1334=ORIENTED_EDGE ( 'NONE', *, *, #2457, .T. ) ;
#1335=VECTOR ( 'NONE', #2052, 1000.000000000000000 ) ;
#1338=CARTESIAN_POINT ( 'NONE',  ( -249.5207023207451300, 1.843143693225357538E-15, 491.2832465756980014 ) ) ;
#1339=DIRECTION ( 'NONE',  ( 0.09383933793885568253, -2.673190762809473730E-31, -0.9955873536034882676 ) ) ;
#1342=ORIENTED_EDGE ( 'NONE', *, *, #2342, .F. ) ;
#1347=DIRECTION ( 'NONE',  ( 1.000000000000000000, 0.000000000000000000, 0.000000000000000000 ) ) ;
#1348=VECTOR ( 'NONE', #176, 1000.000000000000000 ) ;
#1350=CARTESIAN_POINT ( 'NONE',  ( 23.50217280488020677, 5.421010862427522170E-17, 428.9062724124374881 ) ) ;
#1352=TOROIDAL_SURFACE ( 'NONE', #3898, 30.50000000000105516, 1.000000000000000000 ) ;
#1354=DIRECTION ( 'NONE',  ( -0.9955873536034883786, 5.498529991225532086E-31, -0.09383933793885522456 ) ) ;
#1355=CARTESIAN_POINT ( 'NONE',  ( -107.0991749147294172, 1.572093150103981429E-15, 535.0680222229615310 ) ) ;
#1356=CARTESIAN_POINT ( 'NONE',  ( -105.2090356704105147, 2.222614453595284090E-15, 560.1816718768288865 ) ) ;
#1357=FACE_OUTER_BOUND ( 'NONE', #4733, .T. ) ;
#1359=AXIS2_PLACEMENT_3D ( 'NONE', #2253, #3471, #615 ) ;
#1360=AXIS2_PLACEMENT_3D ( 'NONE', #1880, #4089, #1993 ) ;
#1361=ORIENTED_EDGE ( 'NONE', *, *, #1034, .T. ) ;
#1362=ORIENTED_EDGE ( 'NONE', *, *, #1228, .F. ) ;
#1364=AXIS2_PLACEMENT_3D ( 'NONE', #3445, #5020, #437 ) ;
#1365=DIRECTION ( 'NONE',  ( 0.9955873536034882676, 0.000000000000000000, 0.09383933793885600172 ) ) ;
#1367=DIRECTION ( 'NONE',  ( 0.09383933793885536334, -2.626968444144180070E-31, -0.9955873536034882676 ) ) ;
#1372=ADVANCED_FACE ( 'NONE', ( #3271 ), #1090, .T. ) ;
#1373=CARTESIAN_POINT ( 'NONE',  ( 33.59898979596707136, -24.99999999999981881, 384.0431050523492900 ) ) ;
#1374=DIRECTION ( 'NONE',  ( -0.9955873536034887117, 6.307420567868191288E-31, -0.09383933793885125552 ) ) ;
#1375=ADVANCED_FACE ( 'NONE', ( #1987 ), #3715, .F. ) ;
#1376=EDGE_CURVE ( 'NONE', #3842, #4320, #2913, .T. ) ;
#1378=EDGE_LOOP ( 'NONE', ( #2611, #1754, #4716, #1054 ) ) ;
#1380=CARTESIAN_POINT ( 'NONE',  ( -338.5048350180761076, 2.276824562219559311E-15, 38.80891300457378890 ) ) ;
#1381=ORIENTED_EDGE ( 'NONE', *, *, #1471, .T. ) ;
#1382=CARTESIAN_POINT ( 'NONE',  ( -223.9642223310785312, 5.421010862427522170E-17, 534.3227077389987016 ) ) ;
#1383=AXIS2_PLACEMENT_3D ( 'NONE', #1380, #2090, #1666 ) ;
#1384=EDGE_LOOP ( 'NONE', ( #5327, #1507, #1441, #2191 ) ) ;
#1386=CARTESIAN_POINT ( 'NONE',  ( 12.58979647763662513, -25.00000000000000355, 97.46177917735926144 ) ) ;
#1389=CIRCLE ( 'NONE', #2086, 1.000000000000000888 ) ;
#1390=VERTEX_POINT ( 'NONE', #3672 ) ;
#1394=ORIENTED_EDGE ( 'NONE', *, *, #320, .F. ) ;
#1395=CARTESIAN_POINT ( 'NONE',  ( -344.4167133082243595, 2.222614453595284090E-15, 101.5309162815936048 ) ) ;
#1398=VERTEX_POINT ( 'NONE', #341 ) ;
#1399=CARTESIAN_POINT ( 'NONE',  ( -36.58361131987999926, -24.99999999999981881, 532.6725316595209279 ) ) ;
#1400=FACE_OUTER_BOUND ( 'NONE', #3859, .T. ) ;
#1401=EDGE_CURVE ( 'NONE', #3100, #936, #2692, .T. ) ;
#1402=AXIS2_PLACEMENT_3D ( 'NONE', #2873, #32, #3401 ) ;
#1403=EDGE_CURVE ( 'NONE', #5281, #4568, #144, .T. ) ;
#1404=CARTESIAN_POINT ( 'NONE',  ( -379.3436097884102765, 6.080251870909620328E-15, 136.4072965734520153 ) ) ;
#1405=LINE ( 'NONE', #4318, #2081 ) ;
#1406=ORIENTED_EDGE ( 'NONE', *, *, #1156, .T. ) ;
#1407=CARTESIAN_POINT ( 'NONE',  ( -105.2090356704105147, 2.222614453595284090E-15, 560.1816718768288865 ) ) ;
#1410=CARTESIAN_POINT ( 'NONE',  ( -320.6447527397726276, 2.276824562219559311E-15, 453.8399743637901906 ) ) ;
#1411=DIRECTION ( 'NONE',  ( 0.09383933793885568253, -2.673190762809473730E-31, -0.9955873536034882676 ) ) ;
#1412=ORIENTED_EDGE ( 'NONE', *, *, #2648, .T. ) ;
#1413=ORIENTED_EDGE ( 'NONE', *, *, #2066, .F. ) ;
#1417=EDGE_LOOP ( 'NONE', ( #584, #3489, #5139, #173 ) ) ;
#1418=DIRECTION ( 'NONE',  ( 1.000000000000000000, -3.851859888774468203E-31, 0.000000000000000000 ) ) ;
#1419=CARTESIAN_POINT ( 'NONE',  ( 23.50217280488020677, 5.421010862427522170E-17, 428.9062724124374881 ) ) ;
#1421=CIRCLE ( 'NONE', #1504, 27.50000000000126121 ) ;
#1422=CIRCLE ( 'NONE', #4589, 21.00000000000012790 ) ;
#1424=CARTESIAN_POINT ( 'NONE',  ( 5.624351423727398824, 25.00000000000018474, 474.0483466084681368 ) ) ;
#1425=SHAPE_REPRESENTATION_RELATIONSHIP ( 'NONE' , 'NONE' ,  #2334, #2204 ) ;
#1427=CIRCLE ( 'NONE', #3546, 4.382543221487789964 ) ;
#1429=CARTESIAN_POINT ( 'NONE',  ( -36.58361131987999926, 25.00000000000018474, 532.6725316595209279 ) ) ;
#1430=CIRCLE ( 'NONE', #4504, 21.00000000000124700 ) ;
#1431=ORIENTED_EDGE ( 'NONE', *, *, #2648, .F. ) ;
#1433=AXIS2_PLACEMENT_3D ( 'NONE', #3834, #4982, #3429 ) ;
#1435=EDGE_CURVE ( 'NONE', #195, #3013, #328, .T. ) ;
#1438=VERTEX_POINT ( 'NONE', #4915 ) ;
#1441=ORIENTED_EDGE ( 'NONE', *, *, #4555, .T. ) ;
#1442=FACE_BOUND ( 'NONE', #685, .T. ) ;
#1443=DIRECTION ( 'NONE',  ( 0.9955873536034882676, 0.000000000000000000, 0.09383933793885600172 ) ) ;
#1445=AXIS2_PLACEMENT_3D ( 'NONE', #469, #2150, #3421 ) ;
#1446=TOROIDAL_SURFACE ( 'NONE', #1012, 28.50000000000115463, 1.000000000000000000 ) ;
#1447=CIRCLE ( 'NONE', #214, 12.50000000000008704 ) ;
#1448=CARTESIAN_POINT ( 'NONE',  ( -344.4167133082243595, -14.95948628165117178, 101.5309162815936048 ) ) ;
#1452=CARTESIAN_POINT ( 'NONE',  ( -312.0566616799260373, -25.00000000000003197, 419.2731246273838792 ) ) ;
#1454=CARTESIAN_POINT ( 'NONE',  ( -349.8593949086763928, 2.222614453595284090E-15, 159.2749827905956010 ) ) ;
#1456=ADVANCED_FACE ( 'NONE', ( #4892 ), #1960, .T. ) ;
#1457=CARTESIAN_POINT ( 'NONE',  ( 34.60640066538633874, 2.222614453595284090E-15, 295.6817845355787995 ) ) ;
#1460=CARTESIAN_POINT ( 'NONE',  ( 29.77542608467492613, 2.222614453595284090E-15, 249.2409987768030533 ) ) ;
#1461=ORIENTED_EDGE ( 'NONE', *, *, #5021, .T. ) ;
#1463=DIRECTION ( 'NONE',  ( -0.9955873536034883786, 5.452307672560241053E-31, -0.09383933793885559926 ) ) ;
#1465=EDGE_CURVE ( 'NONE', #281, #742, #1235, .T. ) ;
#1466=EDGE_LOOP ( 'NONE', ( #5338, #1334, #4557, #4632 ) ) ;
#1470=CYLINDRICAL_SURFACE ( 'NONE', #910, 4.382543221487789964 ) ;
#1471=EDGE_CURVE ( 'NONE', #4644, #689, #1430, .T. ) ;
#1472=EDGE_LOOP ( 'NONE', ( #4622, #799 ) ) ;
#1475=CARTESIAN_POINT ( 'NONE',  ( 36.66581985038887126, -24.99999999999981881, 340.1662229844756098 ) ) ;
#1478=DIRECTION ( 'NONE',  ( -0.09383933793885568253, 2.673190762809473730E-31, 0.9955873536034882676 ) ) ;
#1479=CARTESIAN_POINT ( 'NONE',  ( 23.50217280488020677, 5.421010862427522170E-17, 428.9062724124374881 ) ) ;
#1481=CARTESIAN_POINT ( 'NONE',  ( -5.157059352427092236, -24.99999999999981881, 435.5986320196304860 ) ) ;
#1482=ORIENTED_EDGE ( 'NONE', *, *, #2888, .F. ) ;
#1483=CARTESIAN_POINT ( 'NONE',  ( -0.4023372602957597799, 1.572093150103981429E-15, 421.4664991284013809 ) ) ;
#1484=ORIENTED_EDGE ( 'NONE', *, *, #3088, .F. ) ;
#1495=FACE_OUTER_BOUND ( 'NONE', #4634, .T. ) ;
#1499=DIRECTION ( 'NONE',  ( -0.09383933793885568253, 2.673190762809473730E-31, 0.9955873536034882676 ) ) ;
#1500=CARTESIAN_POINT ( 'NONE',  ( -320.6447527397726276, 2.276824562219559311E-15, 453.8399743637901906 ) ) ;
#1502=CARTESIAN_POINT ( 'NONE',  ( -299.8611223228758149, 3.740497495074990297E-15, 439.6443911606511392 ) ) ;
#1503=CARTESIAN_POINT ( 'NONE',  ( 16.26935751051944479, 3.252606517456513302E-16, 140.3055424402290896 ) ) ;
#1504=AXIS2_PLACEMENT_3D ( 'NONE', #1027, #4333, #536 ) ;
#1506=CARTESIAN_POINT ( 'NONE',  ( -367.0882437885064746, 25.00000000000018474, 297.8351940652706276 ) ) ;
#1507=ORIENTED_EDGE ( 'NONE', *, *, #5021, .F. ) ;
#1510=DIRECTION ( 'NONE',  ( -0.01527226085271972227, -2.080004339938201146E-31, -0.9998833722232041143 ) ) ;
#1511=CIRCLE ( 'NONE', #3716, 21.00000000000012790 ) ;
#1513=EDGE_CURVE ( 'NONE', #4212, #4831, #612, .T. ) ;
#1514=VECTOR ( 'NONE', #1039, 1000.000000000000000 ) ;
#1519=DIRECTION ( 'NONE',  ( -0.9955873536034883786, 5.498529991225532086E-31, -0.09383933793885522456 ) ) ;
#1520=FACE_OUTER_BOUND ( 'NONE', #1417, .T. ) ;
#1521=STYLED_ITEM('',(#5451),#4977);
#1524=ORIENTED_EDGE ( 'NONE', *, *, #1692, .T. ) ;
#1527=AXIS2_PLACEMENT_3D ( 'NONE', #1320, #754, #2465 ) ;
#1528=CARTESIAN_POINT ( 'NONE',  ( -351.5485029915759583, 2.222614453595284090E-15, 177.1955551554592603 ) ) ;
#1529=DIRECTION ( 'NONE',  ( -0.09383933793885537722, 2.626968444144180508E-31, 0.9955873536034883786 ) ) ;
#1530=AXIS2_PLACEMENT_3D ( 'NONE', #1395, #1824, #2217 ) ;
#1532=CIRCLE ( 'NONE', #652, 4.382543221487789076 ) ;
#1533=AXIS2_PLACEMENT_3D ( 'NONE', #3128, #4792, #2245 ) ;
#1536=FACE_OUTER_BOUND ( 'NONE', #1902, .T. ) ;
#1537=CARTESIAN_POINT ( 'NONE',  ( -107.0991749147297014, 25.00000000000018474, 535.0680222229608489 ) ) ;
#1538=CARTESIAN_POINT ( 'NONE',  ( -36.58361131987999926, -24.99999999999981881, 532.6725316595209279 ) ) ;
#1540=ADVANCED_FACE ( 'NONE', ( #4732, #3825 ), #876, .T. ) ;
#1542=PRODUCT_DEFINITION_FORMATION_WITH_SPECIFIED_SOURCE ( 'ANY', '', #2460, .NOT_KNOWN. ) ;
#1544=CARTESIAN_POINT ( 'NONE',  ( -0.4023372602832280820, 25.00000000000018474, 421.4664991283991640 ) ) ;
#1546=DIRECTION ( 'NONE',  ( 0.09383933793885568253, -2.673190762809473730E-31, -0.9955873536034882676 ) ) ;
#1547=CARTESIAN_POINT ( 'NONE',  ( -346.0119820531830328, 0.000000000000000000, 118.4559012928528858 ) ) ;
#1556=ORIENTED_EDGE ( 'NONE', *, *, #3185, .T. ) ;
#1557=CARTESIAN_POINT ( 'NONE',  ( -351.7361816674535362, 5.421010862427522170E-17, 179.1867298626658283 ) ) ;
#1560=CARTESIAN_POINT ( 'NONE',  ( -334.2354697480813002, 2.276824562219556945E-15, 40.21575531256979019 ) ) ;
#1563=DIRECTION ( 'NONE',  ( -0.09383933793885568253, 2.673190762809473730E-31, 0.9955873536034882676 ) ) ;
#1564=CARTESIAN_POINT ( 'NONE',  ( -213.0979982360508416, 24.99999999999997158, 511.7519955242232754 ) ) ;
#1565=EDGE_CURVE ( 'NONE', #911, #4329, #4225, .T. ) ;
#1566=CARTESIAN_POINT ( 'NONE',  ( -80.60298687151718866, -24.99999999999981881, 555.2885198911441194 ) ) ;
#1568=CARTESIAN_POINT ( 'NONE',  ( 11.65205807320727871, 25.00000000000018474, 340.0738060255407049 ) ) ;
#1570=CIRCLE ( 'NONE', #163, 27.50000000000126121 ) ;
#1573=ORIENTED_EDGE ( 'NONE', *, *, #4793, .T. ) ;
#1574=VERTEX_POINT ( 'NONE', #1694 ) ;
#1575=DIRECTION ( 'NONE',  ( 0.9955873536034882676, -5.499791016784056700E-31, 0.09383933793885550212 ) ) ;
#1578=CYLINDRICAL_SURFACE ( 'NONE', #3372, 21.00000000000124700 ) ;
#1579=FACE_OUTER_BOUND ( 'NONE', #1212, .T. ) ;
#1580=ORIENTED_EDGE ( 'NONE', *, *, #2177, .F. ) ;
#1582=CARTESIAN_POINT ( 'NONE',  ( -364.1439395362591540, 2.222614453595284090E-15, 237.2787335496894343 ) ) ;
#1583=DIRECTION ( 'NONE',  ( -0.9955873536034882676, 5.484003909441380272E-31, -0.09383933793885536334 ) ) ;
#1585=AXIS2_PLACEMENT_3D ( 'NONE', #1956, #362, #2479 ) ;
#1586=DIRECTION ( 'NONE',  ( 0.09383933793885568253, -2.673190762809473730E-31, -0.9955873536034882676 ) ) ;
#1587=CARTESIAN_POINT ( 'NONE',  ( -198.3455225866221667, 24.99999999999997158, 518.3576047634796851 ) ) ;
#1589=CARTESIAN_POINT ( 'NONE',  ( -156.9923520473269321, 0.000000000000000000, 556.8176423728721147 ) ) ;
#1590=ORIENTED_EDGE ( 'NONE', *, *, #4050, .F. ) ;
#1591=CARTESIAN_POINT ( 'NONE',  ( -63.04765821498167355, 25.00000000000018474, 521.0401840782875524 ) ) ;
#1592=ORIENTED_EDGE ( 'NONE', *, *, #1221, .T. ) ;
#1593=DIRECTION ( 'NONE',  ( 0.09383933793885537722, -2.626968444144180508E-31, -0.9955873536034883786 ) ) ;
#1594=FACE_OUTER_BOUND ( 'NONE', #4741, .T. ) ;
#1596=VERTEX_POINT ( 'NONE', #3787 ) ;
#1597=ADVANCED_FACE ( 'NONE', ( #4618 ), #3767, .T. ) ;
#1599=DIRECTION ( 'NONE',  ( 0.09383933793885568253, -2.673190762809473730E-31, -0.9955873536034882676 ) ) ;
#1600=DIRECTION ( 'NONE',  ( -0.9955873536034882676, 5.273458392682099492E-31, -0.09383933793885600172 ) ) ;
#1601=EDGE_CURVE ( 'NONE', #4644, #3314, #81, .T. ) ;
#1605=EDGE_CURVE ( 'NONE', #2877, #3068, #4292, .T. ) ;
#1609=FACE_OUTER_BOUND ( 'NONE', #4336, .T. ) ;
#1610=CARTESIAN_POINT ( 'NONE',  ( -354.3266237013149862, 5.421010862427522170E-17, 381.2801272015580025 ) ) ;
#1613=STYLED_ITEM('',(#5451),#3136);
#1618=CARTESIAN_POINT ( 'NONE',  ( -52.92425795465503313, 25.00000000000018474, 513.6488213284155790 ) ) ;
#1619=CARTESIAN_POINT ( 'NONE',  ( -264.1404626571541598, -25.00000000000003197, 511.7445549721641100 ) ) ;
#1621=CIRCLE ( 'NONE', #1183, 4.382543221487789076 ) ;
#1623=ORIENTED_EDGE ( 'NONE', *, *, #3398, .T. ) ;
#1624=ADVANCED_FACE ( 'NONE', ( #4237, #1724 ), #3391, .F. ) ;
#1627=ORIENTED_EDGE ( 'NONE', *, *, #1787, .F. ) ;
#1632=ORIENTED_EDGE ( 'NONE', *, *, #965, .T. ) ;
#1634=DIRECTION ( 'NONE',  ( -0.9998833722232040033, 6.797399803719615819E-31, 0.01527226085271964420 ) ) ;
#1635=EDGE_CURVE ( 'NONE', #4435, #2041, #2505, .T. ) ;
#1636=FACE_OUTER_BOUND ( 'NONE', #5316, .T. ) ;
#1639=CARTESIAN_POINT ( 'NONE',  ( -86.97194166595129161, 3.740497495074990297E-15, 531.0655262460708173 ) ) ;
#1640=CARTESIAN_POINT ( 'NONE',  ( -13.17877320795229856, 25.00000000000000355, 47.33401081801169141 ) ) ;
#1641=CARTESIAN_POINT ( 'NONE',  ( 35.78913469918423829, 0.000000000000000000, 310.6402212931345161 ) ) ;
#1642=ORIENTED_EDGE ( 'NONE', *, *, #2200, .T. ) ;
#1643=CIRCLE ( 'NONE', #3594, 2.000000000000001776 ) ;
#1645=FACE_OUTER_BOUND ( 'NONE', #2543, .T. ) ;
#1646=AXIS2_PLACEMENT_3D ( 'NONE', #4564, #1586, #789 ) ;
#1647=ORIENTED_EDGE ( 'NONE', *, *, #2888, .T. ) ;
#1648=VERTEX_POINT ( 'NONE', #2945 ) ;
#1652=DIRECTION ( 'NONE',  ( 0.9998833722232041143, -6.779273404243020281E-31, -0.01527226085271993043 ) ) ;
#1653=EDGE_CURVE ( 'NONE', #2041, #4297, #3909, .T. ) ;
#1658=CARTESIAN_POINT ( 'NONE',  ( -17.84624325233685127, 4.358724120770097062E-15, 36.40401889739442254 ) ) ;
#1660=CARTESIAN_POINT ( 'NONE',  ( -320.3751800289425091, 5.421010862425815642E-17, 182.1426690077398689 ) ) ;
#1661=CARTESIAN_POINT ( 'NONE',  ( -342.0244061588616091, 3.740497495074990297E-15, 297.0039604601894894 ) ) ;
#1662=FACE_OUTER_BOUND ( 'NONE', #665, .T. ) ;
#1666=DIRECTION ( 'NONE',  ( -0.9955873536034882676, 5.436595176548168253E-31, -0.09383933793885573804 ) ) ;
#1670=CARTESIAN_POINT ( 'NONE',  ( -353.5191290882918338, 0.000000000000000000, 198.1028895811327573 ) ) ;
#1671=DIRECTION ( 'NONE',  ( -0.9955873536034882676, 5.498529991225543472E-31, -0.09383933793885566865 ) ) ;
#1679=CARTESIAN_POINT ( 'NONE',  ( -377.2791443537555551, 3.911847525938623293E-15, 114.5043747941758596 ) ) ;
#1681=FACE_BOUND ( 'NONE', #3612, .T. ) ;
#1682=CIRCLE ( 'NONE', #4936, 1.000000000000000888 ) ;
#1683=DIRECTION ( 'NONE',  ( -0.9955873536034882676, 0.000000000000000000, -0.09383933793885600172 ) ) ;
#1686=CARTESIAN_POINT ( 'NONE',  ( -23.53079058812344471, -24.99999999999981881, 476.4235034963351154 ) ) ;
#1688=AXIS2_PLACEMENT_3D ( 'NONE', #1874, #1326, #4303 ) ;
#1689=EDGE_CURVE ( 'NONE', #3205, #2195, #5157, .T. ) ;
#1692=EDGE_CURVE ( 'NONE', #463, #276, #1405, .T. ) ;
#1694=CARTESIAN_POINT ( 'NONE',  ( -376.3773963380906480, 1.662953840130941270E-29, 115.5938014857176768 ) ) ;
#1695=AXIS2_PLACEMENT_3D ( 'NONE', #4997, #3393, #1189 ) ;
#1696=EDGE_CURVE ( 'NONE', #4078, #3095, #1114, .T. ) ;
#1697=CIRCLE ( 'NONE', #648, 4.382543221487789964 ) ;
#1701=CARTESIAN_POINT ( 'NONE',  ( -348.7799179161582970, 2.813531315051574489E-15, 101.1196613272007738 ) ) ;
#1703=DIRECTION ( 'NONE',  ( 0.09383933793885568253, -2.673190762809473730E-31, -0.9955873536034882676 ) ) ;
#1706=CARTESIAN_POINT ( 'NONE',  ( -344.1351952944061168, 5.421010862427522170E-17, 98.54415422078321285 ) ) ;
#1707=DIRECTION ( 'NONE',  ( -0.9955873536034882676, 5.498529991225538217E-31, -0.09383933793885536334 ) ) ;
#1709=EDGE_LOOP ( 'NONE', ( #3945, #366 ) ) ;
#1711=ORIENTED_EDGE ( 'NONE', *, *, #1203, .T. ) ;
#1712=DIRECTION ( 'NONE',  ( 0.09383933793885568253, -2.673190762809473730E-31, -0.9955873536034882676 ) ) ;
#1714=DIRECTION ( 'NONE',  ( -0.09383933793885536334, 2.626968444144180070E-31, 0.9955873536034882676 ) ) ;
#1716=ORIENTED_EDGE ( 'NONE', *, *, #1696, .F. ) ;
#1717=ADVANCED_FACE ( 'NONE', ( #4804 ), #2437, .T. ) ;
#1719=CARTESIAN_POINT ( 'NONE',  ( -167.9289969670494997, 3.740497495074990297E-15, 528.5729890193238134 ) ) ;
#1721=ORIENTED_EDGE ( 'NONE', *, *, #1601, .T. ) ;
#1724=FACE_BOUND ( 'NONE', #4138, .T. ) ;
#1727=PLANE ( 'NONE',  #1445 ) ;
#1728=VERTEX_POINT ( 'NONE', #4123 ) ;
#1729=DIRECTION ( 'NONE',  ( 0.09383933793885537722, -2.626968444144180508E-31, -0.9955873536034883786 ) ) ;
#1730=AXIS2_PLACEMENT_3D ( 'NONE', #3109, #2299, #2715 ) ;
#1731=CARTESIAN_POINT ( 'NONE',  ( -342.9618789639491752, 2.813531315051557923E-15, 39.39324540378412109 ) ) ;
#1732=CARTESIAN_POINT ( 'NONE',  ( -121.8424039466566313, 3.794707603699265519E-15, 535.4314447305365547 ) ) ;
#1738=VERTEX_POINT ( 'NONE', #3683 ) ;
#1745=ORIENTED_EDGE ( 'NONE', *, *, #3733, .T. ) ;
#1748=CARTESIAN_POINT ( 'NONE',  ( -86.97194166595193110, -24.99999999999981881, 531.0655262460722952 ) ) ;
#1749=LINE ( 'NONE', #2198, #3473 ) ;
#1750=ORIENTED_EDGE ( 'NONE', *, *, #166, .T. ) ;
#1752=DIRECTION ( 'NONE',  ( -0.9955873536034882676, 5.452307672560245432E-31, -0.09383933793885568253 ) ) ;
#1754=ORIENTED_EDGE ( 'NONE', *, *, #2852, .T. ) ;
#1755=CARTESIAN_POINT ( 'NONE',  ( -80.60298687151650654, 2.222614453595284090E-15, 555.2885198911399129 ) ) ;
#1759=CARTESIAN_POINT ( 'NONE',  ( -213.0979982360508416, -25.00000000000003197, 511.7519955242232754 ) ) ;
#1760=CARTESIAN_POINT ( 'NONE',  ( -333.8864425577414181, 2.759321206427298478E-15, 102.5234496157762578 ) ) ;
#1761=CARTESIAN_POINT ( 'NONE',  ( -324.0724149101815783, 5.421010862424517719E-17, 109.4750664999304348 ) ) ;
#1762=ORIENTED_EDGE ( 'NONE', *, *, #166, .F. ) ;
#1763=ORIENTED_EDGE ( 'NONE', *, *, #4567, .F. ) ;
#1764=ADVANCED_FACE ( 'NONE', ( #5286 ), #3338, .F. ) ;
#1765=ADVANCED_FACE ( 'NONE', ( #1173 ), #4445, .T. ) ;
#1767=CIRCLE ( 'NONE', #5369, 17.00000000000009948 ) ;
#1768=CARTESIAN_POINT ( 'NONE',  ( -374.4800609688232953, 1.553907686679738498E-29, 116.7770675151984392 ) ) ;
#1769=ADVANCED_FACE ( 'NONE', ( #4904 ), #3190, .T. ) ;
#1775=AXIS2_PLACEMENT_3D ( 'NONE', #949, #1051, #5120 ) ;
#1778=CARTESIAN_POINT ( 'NONE',  ( -63.04765821500757284, -24.99999999999981881, 521.0401840782880072 ) ) ;
#1779=DIRECTION ( 'NONE',  ( -0.9955873536034884896, 0.000000000000000000, -0.09383933793885443353 ) ) ;
#1782=AXIS2_PLACEMENT_3D ( 'NONE', #3793, #2919, #344 ) ;
#1787=EDGE_CURVE ( 'NONE', #3984, #5060, #4324, .T. ) ;
#1789=CARTESIAN_POINT ( 'NONE',  ( -264.1404626571534777, 2.222614453595284090E-15, 511.7445549721628595 ) ) ;
#1790=AXIS2_PLACEMENT_3D ( 'NONE', #3942, #193, #3532 ) ;
#1791=CIRCLE ( 'NONE', #2672, 4.382543221487789076 ) ;
#1793=CARTESIAN_POINT ( 'NONE',  ( -0.4023372603089575006, -24.99999999999981881, 421.4664991283988229 ) ) ;
#1794=LINE ( 'NONE', #5266, #2481 ) ;
#1796=VECTOR ( 'NONE', #313, 1000.000000000000114 ) ;
#1801=ORIENTED_EDGE ( 'NONE', *, *, #330, .F. ) ;
#1803=FACE_OUTER_BOUND ( 'NONE', #3535, .T. ) ;
#1804=DIRECTION ( 'NONE',  ( 0.09383933793885537722, -2.626968444144180508E-31, -0.9955873536034883786 ) ) ;
#1805=DIRECTION ( 'NONE',  ( -0.9955873536034883786, 5.498529991225544347E-31, -0.09383933793885444741 ) ) ;
#1809=CARTESIAN_POINT ( 'NONE',  ( -342.0244061588616091, -24.99999999999981881, 297.0039604601892620 ) ) ;
#1811=CARTESIAN_POINT ( 'NONE',  ( -338.5986743560152377, 2.276824562219559311E-15, 39.80450035817695209 ) ) ;
#1812=DIRECTION ( 'NONE',  ( -0.01527226085271972227, -2.080004339938201146E-31, -0.9998833722232041143 ) ) ;
#1814=VERTEX_POINT ( 'NONE', #926 ) ;
#1815=CARTESIAN_POINT ( 'NONE',  ( 18.31346110193259946, 25.00000000000018474, 444.2932575970297648 ) ) ;
#1817=AXIS2_PLACEMENT_3D ( 'NONE', #516, #155, #3521 ) ;
#1819=CARTESIAN_POINT ( 'NONE',  ( 36.66581985038869362, 3.252606517456513302E-16, 340.1662229844753256 ) ) ;
#1821=AXIS2_PLACEMENT_3D ( 'NONE', #3550, #957, #575 ) ;
#1824=DIRECTION ( 'NONE',  ( 0.09383933793885568253, -2.673190762809473730E-31, -0.9955873536034882676 ) ) ;
#1825=CARTESIAN_POINT ( 'NONE',  ( -378.1397951484382816, 2.222614453595299078E-15, 155.6049743057346291 ) ) ;
#1826=DIRECTION ( 'NONE',  ( -0.9955873536034883786, 5.498529991225525955E-31, -0.09383933793885444741 ) ) ;
#1827=FACE_OUTER_BOUND ( 'NONE', #1304, .T. ) ;
#1828=ORIENTED_EDGE ( 'NONE', *, *, #4993, .F. ) ;
#1831=CARTESIAN_POINT ( 'NONE',  ( 16.26935751051938439, -25.00000000000000355, 140.3055424402287770 ) ) ;
#1833=( BOUNDED_SURFACE ( )  B_SPLINE_SURFACE ( 3, 3, ( 
 ( #2179, #3086, #3962, #5218, #1460, #3038, #2641, #5107, #3509, #524, #2206, #1350, #551, #4376, #4709, #3852, #939, #83, #4296, #3481, #2622, #5164, #1755, #1407, #3876, #3914, #4753, #168, #1382, #1789, #110, #3062, #140, #992, #2256, #5138, #3143, #2669 ),
 ( #4734, #4806, #1868, #963, #4321, #189, #501, #3447, #2233, #1841, #2696, #1019, #1815, #4351, #578, #3938, #3529, #5186, #1429, #4785, #1043, #3116, #601, #3555, #2718, #1953, #4454, #277, #3691, #4912, #3640, #4107, #2804, #3256, #3669, #1506, #2366, #1185 ),
 ( #1152, #5326, #3230, #3282, #2336, #3992, #222, #1568, #4946, #3171, #338, #1544, #1067, #2746, #2831, #5268, #3204, #5355, #250, #1591, #660, #3611, #4399, #4865, #684, #4830, #2779, #4019, #4509, #626, #743, #4045, #1924, #1099, #5301, #4889, #1127, #2306 ),
 ( #1985, #4482, #707, #2393, #4077, #2426, #310, #1898, #2010, #3585, #5243, #1483, #4427, #4542, #2866, #768, #2454, #4130, #360, #1251, #3064, #2184, #3004, #1355, #1732, #503, #2598, #4017, #5265, #4736, #1896, #1502, #968, #2624, #113, #2302, #2644, #3199 ),
 ( #3608, #2333, #4677, #2157, #941, #916, #4396, #3426, #4273, #247, #3879, #1793, #1481, #622, #1065, #3169, #3855, #1921, #4243, #5142, #657, #4858, #2561, #5078, #4712, #1322, #3485, #87, #1759, #3450, #4301, #2741, #5110, #478, #3040, #3832, #527, #2210 ),
 ( #63, #1386, #3987, #218, #3583, #5240, #4828, #4424, #2035, #2887, #333, #1096, #3744, #1949, #2775, #1982, #3312, #4042, #1538, #5407, #2475, #2389, #1566, #4566, #4451, #680, #305, #2451, #4972, #1619, #2362, #2424, #4072, #2007, #273, #3689, #1123, #4503 ),
 ( #4910, #738, #3710, #791, #5353, #3636, #1641, #5295, #3227, #3665, #1210, #4886, #2800, #3336, #4155, #5324, #3253, #384, #4479, #704, #1150, #4127, #2061, #2828, #4105, #1589, #3279, #4941, #1180, #2864, #4540, #5381, #764, #358, #2964, #1256, #18, #2552 ) ),
 .UNSPECIFIED., .T., .F., .F. ) 
 B_SPLINE_SURFACE_WITH_KNOTS ( ( 4, 3, 4 ),
 ( 4, 2, 2, 2, 2, 2, 2, 2, 2, 2, 2, 2, 2, 2, 2, 2, 2, 2, 4 ),
 ( 0.000000000000000000, 0.5000000000000000000, 1.000000000000000000 ),
 ( 0.000000000000000000, 0.1028767157186024211, 0.2057534314372048423, 0.2571917892965060459, 0.3086301471558072773, 0.3600685050151084532, 0.4115068628744096846, 0.4558387458985032614, 0.4780046874105500776, 0.5001706289225968938, 0.5231687412733679876, 0.5461668536241390814, 0.5921630783256812691, 0.6381593030272234568, 0.6841555277287657555, 0.7631166457965743444, 0.8420777638643828222, 0.9210388819321914111, 1.000000000000000000 ),
 .UNSPECIFIED. ) 
 GEOMETRIC_REPRESENTATION_ITEM ( )  RATIONAL_B_SPLINE_SURFACE ( (
 ( 1.000000000000000000, 1.000000000000000000, 1.000000000000000000, 1.000000000000000000, 1.000000000000000000, 1.000000000000000000, 1.000000000000000000, 1.000000000000000000, 1.000000000000000000, 1.000000000000000000, 1.000000000000000000, 1.000000000000000000, 1.000000000000000000, 1.000000000000000000, 1.000000000000000000, 1.000000000000000000, 1.000000000000000000, 1.000000000000000000, 1.000000000000000000, 1.000000000000000000, 1.000000000000000000, 1.000000000000000000, 1.000000000000000000, 1.000000000000000000, 1.000000000000000000, 1.000000000000000000, 1.000000000000000000, 1.000000000000000000, 1.000000000000000000, 1.000000000000000000, 1.000000000000000000, 1.000000000000000000, 1.000000000000000000, 1.000000000000000000, 1.000000000000000000, 1.000000000000000000, 1.000000000000000000, 1.000000000000000000),
 ( 0.3333333333333333703, 0.3333333333333333703, 0.3333333333333333703, 0.3333333333333333703, 0.3333333333333333703, 0.3333333333333333703, 0.3333333333333333703, 0.3333333333333333703, 0.3333333333333333703, 0.3333333333333333703, 0.3333333333333333703, 0.3333333333333333703, 0.3333333333333333703, 0.3333333333333333703, 0.3333333333333333703, 0.3333333333333333703, 0.3333333333333333703, 0.3333333333333333703, 0.3333333333333333703, 0.3333333333333333703, 0.3333333333333333703, 0.3333333333333333703, 0.3333333333333333703, 0.3333333333333333703, 0.3333333333333333703, 0.3333333333333333703, 0.3333333333333333703, 0.3333333333333333703, 0.3333333333333333703, 0.3333333333333333703, 0.3333333333333333703, 0.3333333333333333703, 0.3333333333333333703, 0.3333333333333333703, 0.3333333333333333703, 0.3333333333333333703, 0.3333333333333333703, 0.3333333333333333703),
 ( 0.3333333333333333703, 0.3333333333333333703, 0.3333333333333333703, 0.3333333333333333703, 0.3333333333333333703, 0.3333333333333333703, 0.3333333333333333703, 0.3333333333333333703, 0.3333333333333333703, 0.3333333333333333703, 0.3333333333333333703, 0.3333333333333333703, 0.3333333333333333703, 0.3333333333333333703, 0.3333333333333333703, 0.3333333333333333703, 0.3333333333333333703, 0.3333333333333333703, 0.3333333333333333703, 0.3333333333333333703, 0.3333333333333333703, 0.3333333333333333703, 0.3333333333333333703, 0.3333333333333333703, 0.3333333333333333703, 0.3333333333333333703, 0.3333333333333333703, 0.3333333333333333703, 0.3333333333333333703, 0.3333333333333333703, 0.3333333333333333703, 0.3333333333333333703, 0.3333333333333333703, 0.3333333333333333703, 0.3333333333333333703, 0.3333333333333333703, 0.3333333333333333703, 0.3333333333333333703),
 ( 1.000000000000000000, 1.000000000000000000, 1.000000000000000000, 1.000000000000000000, 1.000000000000000000, 1.000000000000000000, 1.000000000000000000, 1.000000000000000000, 1.000000000000000000, 1.000000000000000000, 1.000000000000000000, 1.000000000000000000, 1.000000000000000000, 1.000000000000000000, 1.000000000000000000, 1.000000000000000000, 1.000000000000000000, 1.000000000000000000, 1.000000000000000000, 1.000000000000000000, 1.000000000000000000, 1.000000000000000000, 1.000000000000000000, 1.000000000000000000, 1.000000000000000000, 1.000000000000000000, 1.000000000000000000, 1.000000000000000000, 1.000000000000000000, 1.000000000000000000, 1.000000000000000000, 1.000000000000000000, 1.000000000000000000, 1.000000000000000000, 1.000000000000000000, 1.000000000000000000, 1.000000000000000000, 1.000000000000000000),
 ( 0.3333333333333333703, 0.3333333333333333703, 0.3333333333333333703, 0.3333333333333333703, 0.3333333333333333703, 0.3333333333333333703, 0.3333333333333333703, 0.3333333333333333703, 0.3333333333333333703, 0.3333333333333333703, 0.3333333333333333703, 0.3333333333333333703, 0.3333333333333333703, 0.3333333333333333703, 0.3333333333333333703, 0.3333333333333333703, 0.3333333333333333703, 0.3333333333333333703, 0.3333333333333333703, 0.3333333333333333703, 0.3333333333333333703, 0.3333333333333333703, 0.3333333333333333703, 0.3333333333333333703, 0.3333333333333333703, 0.3333333333333333703, 0.3333333333333333703, 0.3333333333333333703, 0.3333333333333333703, 0.3333333333333333703, 0.3333333333333333703, 0.3333333333333333703, 0.3333333333333333703, 0.3333333333333333703, 0.3333333333333333703, 0.3333333333333333703, 0.3333333333333333703, 0.3333333333333333703),
 ( 0.3333333333333333703, 0.3333333333333333703, 0.3333333333333333703, 0.3333333333333333703, 0.3333333333333333703, 0.3333333333333333703, 0.3333333333333333703, 0.3333333333333333703, 0.3333333333333333703, 0.3333333333333333703, 0.3333333333333333703, 0.3333333333333333703, 0.3333333333333333703, 0.3333333333333333703, 0.3333333333333333703, 0.3333333333333333703, 0.3333333333333333703, 0.3333333333333333703, 0.3333333333333333703, 0.3333333333333333703, 0.3333333333333333703, 0.3333333333333333703, 0.3333333333333333703, 0.3333333333333333703, 0.3333333333333333703, 0.3333333333333333703, 0.3333333333333333703, 0.3333333333333333703, 0.3333333333333333703, 0.3333333333333333703, 0.3333333333333333703, 0.3333333333333333703, 0.3333333333333333703, 0.3333333333333333703, 0.3333333333333333703, 0.3333333333333333703, 0.3333333333333333703, 0.3333333333333333703),
 ( 1.000000000000000000, 1.000000000000000000, 1.000000000000000000, 1.000000000000000000, 1.000000000000000000, 1.000000000000000000, 1.000000000000000000, 1.000000000000000000, 1.000000000000000000, 1.000000000000000000, 1.000000000000000000, 1.000000000000000000, 1.000000000000000000, 1.000000000000000000, 1.000000000000000000, 1.000000000000000000, 1.000000000000000000, 1.000000000000000000, 1.000000000000000000, 1.000000000000000000, 1.000000000000000000, 1.000000000000000000, 1.000000000000000000, 1.000000000000000000, 1.000000000000000000, 1.000000000000000000, 1.000000000000000000, 1.000000000000000000, 1.000000000000000000, 1.000000000000000000, 1.000000000000000000, 1.000000000000000000, 1.000000000000000000, 1.000000000000000000, 1.000000000000000000, 1.000000000000000000, 1.000000000000000000, 1.000000000000000000) ) ) 
 REPRESENTATION_ITEM ( '' )  SURFACE ( )  );
#1836=CARTESIAN_POINT ( 'NONE',  ( 36.66581985038887126, 25.00000000000018474, 340.1662229844756098 ) ) ;
#1841=CARTESIAN_POINT ( 'NONE',  ( 33.59898979596707136, 25.00000000000018474, 384.0431050523492900 ) ) ;
#1842=ORIENTED_EDGE ( 'NONE', *, *, #1946, .F. ) ;
#1844=PLANE ( 'NONE',  #3472 ) ;
#1845=CIRCLE ( 'NONE', #4745, 4.382543221487789076 ) ;
#1847=EDGE_LOOP ( 'NONE', ( #769, #2593 ) ) ;
#1848=DIRECTION ( 'NONE',  ( 0.01527226085271977431, 2.087708059715749652E-31, 0.9998833722232041143 ) ) ;
#1852=ORIENTED_EDGE ( 'NONE', *, *, #4380, .T. ) ;
#1856=CARTESIAN_POINT ( 'NONE',  ( -49.96441683051492078, -24.99999999999981881, 542.4422122871054626 ) ) ;
#1862=CARTESIAN_POINT ( 'NONE',  ( -349.7655555707380017, 2.222614453595284090E-15, 158.2793954369929850 ) ) ;
#1863=CARTESIAN_POINT ( 'NONE',  ( -30.63277980166709114, 25.00000000000018474, 527.1358351633700750 ) ) ;
#1867=EDGE_LOOP ( 'NONE', ( #371, #2172 ) ) ;
#1868=CARTESIAN_POINT ( 'NONE',  ( 16.26935751051938439, 25.00000000000000355, 140.3055424402287770 ) ) ;
#1871=ADVANCED_FACE ( 'NONE', ( #489 ), #2902, .T. ) ;
#1872=DIRECTION ( 'NONE',  ( 0.09383933793885568253, -2.673190762809473730E-31, -0.9955873536034882676 ) ) ;
#1874=CARTESIAN_POINT ( 'NONE',  ( -347.8887688119603467, 2.222614453595284090E-15, 138.3676483649222178 ) ) ;
#1875=CIRCLE ( 'NONE', #5025, 1.000000000000000888 ) ;
#1876=EDGE_LOOP ( 'NONE', ( #2893, #3939 ) ) ;
#1879=CARTESIAN_POINT ( 'NONE',  ( -365.8191009029663974, 5.636683259291067391E-15, 36.23439996194950652 ) ) ;
#1880=CARTESIAN_POINT ( 'NONE',  ( -347.7949294740212736, 2.222614453595284090E-15, 137.3720610113191469 ) ) ;
#1884=CIRCLE ( 'NONE', #4955, 27.50000000000126832 ) ;
#1886=ORIENTED_EDGE ( 'NONE', *, *, #728, .F. ) ;
#1888=( NAMED_UNIT ( * ) SI_UNIT ( $, .STERADIAN. ) SOLID_ANGLE_UNIT ( ) );
#1889=DIRECTION ( 'NONE',  ( -5.679099018122554920E-31, -1.000000000000000000, 2.149753974990777610E-31 ) ) ;
#1890=CARTESIAN_POINT ( 'NONE',  ( 5.624351423727398824, -24.99999999999981881, 474.0483466084681368 ) ) ;
#1893=CARTESIAN_POINT ( 'NONE',  ( -349.7655555707380017, 2.222614453595284090E-15, 158.2793954369929850 ) ) ;
#1894=DIRECTION ( 'NONE',  ( -0.9998833722232040033, 6.797399803719615819E-31, 0.01527226085271964420 ) ) ;
#1896=CARTESIAN_POINT ( 'NONE',  ( -268.5984117390374877, 3.740497495074990297E-15, 475.6392848759629715 ) ) ;
#1898=CARTESIAN_POINT ( 'NONE',  ( 11.65205807320734976, 3.740497495074990297E-15, 340.0738060255405912 ) ) ;
#1902=EDGE_LOOP ( 'NONE', ( #583, #3455, #4112, #1482 ) ) ;
#1903=VERTEX_POINT ( 'NONE', #3737 ) ;
#1904=CARTESIAN_POINT ( 'NONE',  ( -321.4851553309757151, 5.712857831165392007E-15, 161.9494039218531043 ) ) ;
#1909=AXIS2_PLACEMENT_3D ( 'NONE', #1557, #5285, #4063 ) ;
#1911=ORIENTED_EDGE ( 'NONE', *, *, #4038, .F. ) ;
#1912=AXIS2_PLACEMENT_3D ( 'NONE', #3579, #5237, #3166 ) ;
#1913=DIRECTION ( 'NONE',  ( 0.9955873536034882676, -5.273458392682099492E-31, 0.09383933793885600172 ) ) ;
#1914=CARTESIAN_POINT ( 'NONE',  ( -367.0460729392618191, -24.99999999999981881, 268.0688838304706678 ) ) ;
#1915=DIRECTION ( 'NONE',  ( 0.01527226085271972227, 2.095411779493299033E-31, 0.9998833722232041143 ) ) ;
#1917=EDGE_CURVE ( 'NONE', #4985, #3013, #2523, .T. ) ;
#1919=CARTESIAN_POINT ( 'NONE',  ( 12.58979647763672283, 2.222614453595284090E-15, 97.46177917736021357 ) ) ;
#1921=CARTESIAN_POINT ( 'NONE',  ( -48.20943979674346735, -24.99999999999981881, 509.2978244404901602 ) ) ;
#1922=CARTESIAN_POINT ( 'NONE',  ( 24.85474708473287109, 3.252606517456513302E-16, 216.1905617304896623 ) ) ;
#1923=ORIENTED_EDGE ( 'NONE', *, *, #1376, .F. ) ;
#1924=CARTESIAN_POINT ( 'NONE',  ( -312.0566616799260373, 24.99999999999997158, 419.2731246273838792 ) ) ;
#1928=ADVANCED_FACE ( 'NONE', ( #1636 ), #2958, .T. ) ;
#1929=ORIENTED_EDGE ( 'NONE', *, *, #5256, .F. ) ;
#1931=CARTESIAN_POINT ( 'NONE',  ( -320.4162772499240077, -1.001483571081362644E-29, 139.9526428046378044 ) ) ;
#1932=CARTESIAN_POINT ( 'NONE',  ( -338.5048350180761076, 2.276824562219559311E-15, 38.80891300457378890 ) ) ;
#1937=VERTEX_POINT ( 'NONE', #2571 ) ;
#1939=ADVANCED_FACE ( 'NONE', ( #4178 ), #4235, .T. ) ;
#1944=DIRECTION ( 'NONE',  ( -0.9955873536034882676, 5.498529991225532962E-31, -0.09383933793885550212 ) ) ;
#1946=EDGE_CURVE ( 'NONE', #3835, #3650, #2100, .T. ) ;
#1948=CARTESIAN_POINT ( 'NONE',  ( -80.59222536594943165, 25.00000000000018474, 529.1597157429057461 ) ) ;
#1949=CARTESIAN_POINT ( 'NONE',  ( 5.624351423727398824, -24.99999999999981881, 474.0483466084681368 ) ) ;
#1951=CIRCLE ( 'NONE', #3623, 28.50000000000127898 ) ;
#1952=ORIENTED_EDGE ( 'NONE', *, *, #2647, .T. ) ;
#1953=CARTESIAN_POINT ( 'NONE',  ( -156.9923520473274721, 25.00000000000018474, 556.8176423728723421 ) ) ;
#1955=AXIS2_PLACEMENT_3D ( 'NONE', #2434, #4959, #3677 ) ;
#1956=CARTESIAN_POINT ( 'NONE',  ( -0.6802310551622114954, 2.222614453595284090E-15, 47.14310755735262859 ) ) ;
#1958=AXIS2_PLACEMENT_3D ( 'NONE', #5052, #4242, #1296 ) ;
#1959=EDGE_CURVE ( 'NONE', #744, #3745, #1069, .T. ) ;
#1960=TOROIDAL_SURFACE ( 'NONE', #2662, 30.50000000000110845, 1.000000000000000000 ) ;
#1964=ORIENTED_EDGE ( 'NONE', *, *, #1376, .T. ) ;
#1965=CARTESIAN_POINT ( 'NONE',  ( -351.6423423295148041, 5.421010862427522170E-17, 178.1911425090623311 ) ) ;
#1969=TOROIDAL_SURFACE ( 'NONE', #3728, 28.50000000000115818, 1.000000000000000000 ) ;
#1970=CARTESIAN_POINT ( 'NONE',  ( -338.5986743560152377, -14.95948628165117178, 39.80450035817695209 ) ) ;
#1971=ORIENTED_EDGE ( 'NONE', *, *, #275, .T. ) ;
#1974=AXIS2_PLACEMENT_3D ( 'NONE', #3415, #872, #3845 ) ;
#1976=CARTESIAN_POINT ( 'NONE',  ( -322.4807426845795817, 2.222614453595269496E-15, 161.8555645839142016 ) ) ;
#1981=CARTESIAN_POINT ( 'NONE',  ( 11.65205807320727871, 25.00000000000018474, 340.0738060255407049 ) ) ;
#1982=CARTESIAN_POINT ( 'NONE',  ( -14.89480152442222582, -24.99999999999981881, 508.6517828409982940 ) ) ;
#1985=CARTESIAN_POINT ( 'NONE',  ( -13.17877320795268759, 1.897353801849632760E-15, 47.33401081801291355 ) ) ;
#1986=ORIENTED_EDGE ( 'NONE', *, *, #792, .F. ) ;
#1987=FACE_OUTER_BOUND ( 'NONE', #3292, .T. ) ;
#1991=ORIENTED_EDGE ( 'NONE', *, *, #2250, .F. ) ;
#1992=CYLINDRICAL_SURFACE ( 'NONE', #4938, 22.67218956682437536 ) ;
#1993=DIRECTION ( 'NONE',  ( -0.9955873536034881566, 5.462637660443544243E-31, -0.09383933793885600172 ) ) ;
#1995=CARTESIAN_POINT ( 'NONE',  ( -340.0535087002904220, 14.95948628165116823, 101.9421712359864500 ) ) ;
#1998=DIRECTION ( 'NONE',  ( -0.9998833722232040033, 6.797399803719615819E-31, 0.01527226085271964420 ) ) ;
#1999=DIRECTION ( 'NONE',  ( -0.9955873536034882676, 5.502656983963329947E-31, -0.09383933793885568253 ) ) ;
#2000=CARTESIAN_POINT ( 'NONE',  ( -338.5048350180761076, 2.276824562219559311E-15, 38.80891300457378890 ) ) ;
#2001=CARTESIAN_POINT ( 'NONE',  ( -351.6423423295148041, 5.421010862427522170E-17, 178.1911425090623311 ) ) ;
#2004=DIRECTION ( 'NONE',  ( 1.000000000000000000, -5.720779902258398713E-31, 0.000000000000000000 ) ) ;
#2005=CARTESIAN_POINT ( 'NONE',  ( -36.58361131987999926, 25.00000000000018474, 532.6725316595209279 ) ) ;
#2007=CARTESIAN_POINT ( 'NONE',  ( -354.3266237013165778, -24.99999999999981881, 381.2801272015587983 ) ) ;
#2008=EDGE_CURVE ( 'NONE', #1438, #4669, #1421, .T. ) ;
#2009=ORIENTED_EDGE ( 'NONE', *, *, #1959, .T. ) ;
#2010=CARTESIAN_POINT ( 'NONE',  ( 11.35554381053716000, 3.794707603699265519E-15, 353.5846600851142512 ) ) ;
#2012=ADVANCED_FACE ( 'NONE', ( #95 ), #5099, .F. ) ;
#2013=EDGE_CURVE ( 'NONE', #1574, #744, #4837, .T. ) ;
#2014=DIRECTION ( 'NONE',  ( -0.9955873536034882676, 5.452307672560241053E-31, -0.09383933793885547436 ) ) ;
#2016=DIRECTION ( 'NONE',  ( 0.09383933793885568253, -2.673190762809473730E-31, -0.9955873536034882676 ) ) ;
#2023=DIRECTION ( 'NONE',  ( -0.9955873536034882676, 5.273458392682099492E-31, -0.09383933793885600172 ) ) ;
#2024=DIRECTION ( 'NONE',  ( -0.9955873536034882676, 5.273458392682099492E-31, -0.09383933793885600172 ) ) ;
#2025=ORIENTED_EDGE ( 'NONE', *, *, #4925, .T. ) ;
#2026=ORIENTED_EDGE ( 'NONE', *, *, #1959, .F. ) ;
#2028=CARTESIAN_POINT ( 'NONE',  ( -80.60298687151650654, 2.222614453595284090E-15, 555.2885198911399129 ) ) ;
#2030=ADVANCED_FACE ( 'NONE', ( #3492 ), #2733, .T. ) ;
#2031=EDGE_CURVE ( 'NONE', #3095, #4078, #1767, .T. ) ;
#2032=CARTESIAN_POINT ( 'NONE',  ( -353.5191290882918338, 0.000000000000000000, 198.1028895811323025 ) ) ;
#2033=DIRECTION ( 'NONE',  ( 0.09383933793885568253, -2.673190762809473730E-31, -0.9955873536034882676 ) ) ;
#2034=CARTESIAN_POINT ( 'NONE',  ( 11.35554381052501682, 25.00000000000018474, 353.5846600851141943 ) ) ;
#2035=CARTESIAN_POINT ( 'NONE',  ( 36.35777514575907787, -24.99999999999981881, 354.7349908125917750 ) ) ;
#2036=ORIENTED_EDGE ( 'NONE', *, *, #1230, .T. ) ;
#2038=DIRECTION ( 'NONE',  ( -0.9955873536034882676, 5.498529991225532086E-31, -0.09383933793885536334 ) ) ;
#2039=DIRECTION ( 'NONE',  ( -0.9955873536034882676, 5.456801509096968857E-31, -0.09383933793885568253 ) ) ;
#2041=VERTEX_POINT ( 'NONE', #1825 ) ;
#2043=VECTOR ( 'NONE', #5278, 1000.000000000000000 ) ;
#2044=DIRECTION ( 'NONE',  ( -1.219242865862094703E-16, 1.000000000000000000, -1.149200448409285278E-17 ) ) ;
#2046=CYLINDRICAL_SURFACE ( 'NONE', #3810, 31.50000000000125766 ) ;
#2049=AXIS2_PLACEMENT_3D ( 'NONE', #2724, #4405, #637 ) ;
#2052=DIRECTION ( 'NONE',  ( 0.01527226085271972227, 2.095411779493299033E-31, 0.9998833722232041143 ) ) ;
#2053=AXIS2_PLACEMENT_3D ( 'NONE', #5343, #2378, #3216 ) ;
#2059=CARTESIAN_POINT ( 'NONE',  ( 8.821273309647297722, 3.740497495074990297E-15, 380.5076279642372015 ) ) ;
#2060=CARTESIAN_POINT ( 'NONE',  ( -63.04765821498167355, 25.00000000000018474, 521.0401840782875524 ) ) ;
#2061=CARTESIAN_POINT ( 'NONE',  ( -80.60298687151650654, 2.222614453595284090E-15, 555.2885198911399129 ) ) ;
#2062=AXIS2_PLACEMENT_3D ( 'NONE', #1038, #3135, #2690 ) ;
#2063=AXIS2_PLACEMENT_3D ( 'NONE', #4028, #5340, #3214 ) ;
#2066=EDGE_CURVE ( 'NONE', #4617, #5050, #2911, .T. ) ;
#2067=DIRECTION ( 'NONE',  ( -0.9955873536034882676, 5.436595176548168253E-31, -0.09383933793885573804 ) ) ;
#2069=ORIENTED_EDGE ( 'NONE', *, *, #5256, .T. ) ;
#2070=DIRECTION ( 'NONE',  ( -0.9955873536034886007, 6.162975822039140717E-31, -0.09383933793885225472 ) ) ;
#2071=CARTESIAN_POINT ( 'NONE',  ( -329.5232379498077080, 5.421010862427522170E-17, 102.9347045701690604 ) ) ;
#2076=ORIENTED_EDGE ( 'NONE', *, *, #2008, .T. ) ;
#2080=CARTESIAN_POINT ( 'NONE',  ( -353.5191290882918338, 0.000000000000000000, 198.1028895811323025 ) ) ;
#2081=VECTOR ( 'NONE', #620, 1000.000000000000114 ) ;
#2082=CYLINDRICAL_SURFACE ( 'NONE', #3291, 12.50000000000003197 ) ;
#2083=CARTESIAN_POINT ( 'NONE',  ( -39.32426838448843398, 3.740497495074990297E-15, 499.4571537926191240 ) ) ;
#2084=CARTESIAN_POINT ( 'NONE',  ( -339.2542556961722084, 3.740497495074990297E-15, 239.6247169981598972 ) ) ;
#2086=AXIS2_PLACEMENT_3D ( 'NONE', #2292, #5154, #2635 ) ;
#2087=VERTEX_POINT ( 'NONE', #5229 ) ;
#2089=CIRCLE ( 'NONE', #1821, 12.50000000000009237 ) ;
#2090=DIRECTION ( 'NONE',  ( 0.09383933793885568253, -2.673190762809473730E-31, -0.9955873536034882676 ) ) ;
#2095=CARTESIAN_POINT ( 'NONE',  ( -342.9618789639491752, -14.95948628165117178, 39.39324540378412109 ) ) ;
#2096=CARTESIAN_POINT ( 'NONE',  ( -380.0371305177060322, 3.252606517456679456E-16, 154.4217082762537245 ) ) ;
#2097=ORIENTED_EDGE ( 'NONE', *, *, #695, .T. ) ;
#2099=DIRECTION ( 'NONE',  ( -0.01527226085271972227, -2.080004339938201146E-31, -0.9998833722232041143 ) ) ;
#2100=LINE ( 'NONE', #2193, #5272 ) ;
#2102=EDGE_CURVE ( 'NONE', #2695, #4403, #1951, .T. ) ;
#2104=DIRECTION ( 'NONE',  ( 0.9955873536034883786, -5.498529991225525955E-31, 0.09383933793885444741 ) ) ;
#2106=ADVANCED_FACE ( 'NONE', ( #3947 ), #3538, .T. ) ;
#2107=CARTESIAN_POINT ( 'NONE',  ( -349.6717162327985307, 3.252606517456513302E-16, 157.2838080833889194 ) ) ;
#2108=CARTESIAN_POINT ( 'NONE',  ( -23.53079058812296154, 3.740497495074990297E-15, 476.4235034963361954 ) ) ;
#2113=CARTESIAN_POINT ( 'NONE',  ( -338.5048350180761076, 2.276824562219559311E-15, 38.80891300457378890 ) ) ;
#2118=CARTESIAN_POINT ( 'NONE',  ( -381.0327178713096714, 6.080251870909624272E-15, 154.3278689383148503 ) ) ;
#2119=DIRECTION ( 'NONE',  ( -0.09383933793885568253, 2.673190762809473730E-31, 0.9955873536034882676 ) ) ;
#2120=CARTESIAN_POINT ( 'NONE',  ( -376.4176382211731493, 1.317201266864838728E-29, 195.9445848085386217 ) ) ;
#2121=CYLINDRICAL_SURFACE ( 'NONE', #1163, 17.00000000000009948 ) ;
#2126=VERTEX_POINT ( 'NONE', #4839 ) ;
#2129=CARTESIAN_POINT ( 'NONE',  ( -347.7949294740212736, 2.222614453595284090E-15, 137.3720610113191469 ) ) ;
#2131=CARTESIAN_POINT ( 'NONE',  ( -342.9618789639491752, 14.95948628165116823, 39.39324540378412109 ) ) ;
#2139=CARTESIAN_POINT ( 'NONE',  ( -23.53079058812296154, 3.740497495074990297E-15, 476.4235034963361954 ) ) ;
#2140=AXIS2_PLACEMENT_3D ( 'NONE', #951, #2220, #3896 ) ;
#2141=CARTESIAN_POINT ( 'NONE',  ( -107.0991749147294172, 1.572093150103981429E-15, 535.0680222229615310 ) ) ;
#2143=AXIS2_PLACEMENT_3D ( 'NONE', #1236, #2016, #4647 ) ;
#2146=EDGE_LOOP ( 'NONE', ( #2036, #1964, #3011, #3872 ) ) ;
#2150=DIRECTION ( 'NONE',  ( 0.09383933793885568253, -2.673190762809473730E-31, -0.9955873536034882676 ) ) ;
#2152=CYLINDRICAL_SURFACE ( 'NONE', #3811, 22.67218956682437536 ) ;
#2155=DIRECTION ( 'NONE',  ( -0.9955873536034882676, 5.456801509096969733E-31, -0.09383933793885547436 ) ) ;
#2157=CARTESIAN_POINT ( 'NONE',  ( 0.07030049708446614587, -25.00000000000000355, 219.5055207296742026 ) ) ;
#2159=DIRECTION ( 'NONE',  ( 0.09383933793885537722, -2.626968444144180508E-31, -0.9955873536034883786 ) ) ;
#2164=ORIENTED_EDGE ( 'NONE', *, *, #4862, .T. ) ;
#2165=CARTESIAN_POINT ( 'NONE',  ( -365.8870837615305618, 2.625968386833868739E-15, 105.5338143064982717 ) ) ;
#2169=CARTESIAN_POINT ( 'NONE',  ( -121.8424039466566313, 3.794707603699265519E-15, 535.4314447305365547 ) ) ;
#2170=CARTESIAN_POINT ( 'NONE',  ( -16.96312831416352296, 1.572093150103981429E-15, 463.2830513152439380 ) ) ;
#2172=ORIENTED_EDGE ( 'NONE', *, *, #1689, .F. ) ;
#2174=DIRECTION ( 'NONE',  ( 0.09383933793885568253, -2.673190762809473730E-31, -0.9955873536034882676 ) ) ;
#2175=EDGE_CURVE ( 'NONE', #742, #3068, #459, .T. ) ;
#2177=EDGE_CURVE ( 'NONE', #3314, #2087, #378, .T. ) ;
#2179=CARTESIAN_POINT ( 'NONE',  ( 11.81831109762787690, 2.222614453595284090E-15, 46.95220429669389262 ) ) ;
#2180=ADVANCED_FACE ( 'NONE', ( #4439 ), #639, .T. ) ;
#2181=CIRCLE ( 'NONE', #5241, 1.000000000000000888 ) ;
#2184=CARTESIAN_POINT ( 'NONE',  ( -80.59222536594906217, 3.740497495074990297E-15, 529.1597157429033587 ) ) ;
#2185=CARTESIAN_POINT ( 'NONE',  ( -367.0460729392618759, 0.000000000000000000, 268.0688838304710089 ) ) ;
#2187=AXIS2_PLACEMENT_3D ( 'NONE', #3251, #1499, #4069 ) ;
#2189=ORIENTED_EDGE ( 'NONE', *, *, #4096, .T. ) ;
#2191=ORIENTED_EDGE ( 'NONE', *, *, #2175, .F. ) ;
#2192=LINE ( 'NONE', #94, #2416 ) ;
#2193=CARTESIAN_POINT ( 'NONE',  ( -349.1289451064980085, 2.222614453595281723E-15, 38.81196702399444121 ) ) ;
#2195=VERTEX_POINT ( 'NONE', #2377 ) ;
#2197=CARTESIAN_POINT ( 'NONE',  ( -39.32426838448843398, 3.740497495074990297E-15, 499.4571537926191240 ) ) ;
#2198=CARTESIAN_POINT ( 'NONE',  ( -312.7741936558949760, 5.421010862425789758E-17, 101.5000933658572677 ) ) ;
#2199=EDGE_CURVE ( 'NONE', #5060, #3984, #545, .T. ) ;
#2200=EDGE_CURVE ( 'NONE', #3237, #4329, #5342, .T. ) ;
#2204=ADVANCED_BREP_SHAPE_REPRESENTATION ( '', ( #4927, #4977, #1285, #3136, #2926 ), #5309 ) ;
#2206=CARTESIAN_POINT ( 'NONE',  ( 31.14585677005082687, 2.222614453595284090E-15, 398.7793066466531968 ) ) ;
#2207=EDGE_CURVE ( 'NONE', #4277, #2126, #1422, .T. ) ;
#2208=EDGE_CURVE ( 'NONE', #2943, #3490, #2222, .T. ) ;
#2209=CARTESIAN_POINT ( 'NONE',  ( -349.6717162327985307, 3.252606517456513302E-16, 157.2838080833889194 ) ) ;
#2210=CARTESIAN_POINT ( 'NONE',  ( -339.2542556961734590, -24.99999999999981881, 239.6247169981589309 ) ) ;
#2211=CARTESIAN_POINT ( 'NONE',  ( -354.3266237013149862, 5.421010862427522170E-17, 381.2801272015580025 ) ) ;
#2212=CARTESIAN_POINT ( 'NONE',  ( -324.1698507674790335, 2.222614453595274229E-15, 179.7761369487778609 ) ) ;
#2214=EDGE_LOOP ( 'NONE', ( #1852, #3085, #952, #4266 ) ) ;
#2215=ORIENTED_EDGE ( 'NONE', *, *, #2177, .T. ) ;
#2217=DIRECTION ( 'NONE',  ( -0.9955873536034882676, 5.452307672560245432E-31, -0.09383933793885568253 ) ) ;
#2220=DIRECTION ( 'NONE',  ( 0.09383933793885537722, -2.626968444144180508E-31, -0.9955873536034883786 ) ) ;
#2221=ORIENTED_EDGE ( 'NONE', *, *, #3615, .F. ) ;
#2222=CIRCLE ( 'NONE', #903, 4.382543221487789076 ) ;
#2223=CYLINDRICAL_SURFACE ( 'NONE', #1817, 12.50000000000009237 ) ;
#2224=CARTESIAN_POINT ( 'NONE',  ( 29.77542608467492613, 2.222614453595284090E-15, 249.2409987768030533 ) ) ;
#2225=DIRECTION ( 'NONE',  ( -0.9955873536034882676, 5.436595176548168253E-31, -0.09383933793885573804 ) ) ;
#2226=VECTOR ( 'NONE', #3228, 1000.000000000000000 ) ;
#2229=CARTESIAN_POINT ( 'NONE',  ( 11.81831109762787690, 2.222614453595284090E-15, 46.95220429669389262 ) ) ;
#2232=ORIENTED_EDGE ( 'NONE', *, *, #2207, .F. ) ;
#2233=CARTESIAN_POINT ( 'NONE',  ( 36.35777514575907787, 25.00000000000018474, 354.7349908125917750 ) ) ;
#2238=VECTOR ( 'NONE', #2468, 1000.000000000000000 ) ;
#2239=CARTESIAN_POINT ( 'NONE',  ( -174.3534642324304116, 5.421010862427522170E-17, 552.7876087698471110 ) ) ;
#2245=DIRECTION ( 'NONE',  ( -0.9955873536034882676, 5.456801509096968857E-31, -0.09383933793885568253 ) ) ;
#2246=DIRECTION ( 'NONE',  ( -0.9998833722232040033, 6.797399803719615819E-31, 0.01527226085271964420 ) ) ;
#2248=ORIENTED_EDGE ( 'NONE', *, *, #3821, .T. ) ;
#2250=EDGE_CURVE ( 'NONE', #3339, #2477, #631, .T. ) ;
#2252=CARTESIAN_POINT ( 'NONE',  ( -49.96441683051505578, 2.222614453595284090E-15, 542.4422122871075089 ) ) ;
#2253=CARTESIAN_POINT ( 'NONE',  ( -315.5527284303366855, 5.957787190994857570E-15, 120.3224137463851520 ) ) ;
#2254=EDGE_LOOP ( 'NONE', ( #4278, #3061, #448, #1632 ) ) ;
#2255=ORIENTED_EDGE ( 'NONE', *, *, #792, .T. ) ;
#2256=CARTESIAN_POINT ( 'NONE',  ( -360.7307227603793649, 2.222614453595284090E-15, 354.4373729494858480 ) ) ;
#2260=DIRECTION ( 'NONE',  ( -0.01527226085271972227, -2.080004339938201584E-31, -0.9998833722232041143 ) ) ;
#2262=ORIENTED_EDGE ( 'NONE', *, *, #4226, .F. ) ;
#2265=DIRECTION ( 'NONE',  ( 0.09383933793885568253, -2.673190762809473730E-31, -0.9955873536034882676 ) ) ;
#2268=ORIENTED_EDGE ( 'NONE', *, *, #2524, .F. ) ;
#2269=CIRCLE ( 'NONE', #2970, 27.43532828739476415 ) ;
#2272=CARTESIAN_POINT ( 'NONE',  ( 29.77542608467487995, -25.00000000000000355, 249.2409987768023711 ) ) ;
#2274=EDGE_CURVE ( 'NONE', #1814, #1596, #3973, .T. ) ;
#2277=FACE_BOUND ( 'NONE', #1876, .T. ) ;
#2278=CARTESIAN_POINT ( 'NONE',  ( -1.533280346156948193, 25.00000000000018474, 488.4857301958397784 ) ) ;
#2286=DIRECTION ( 'NONE',  ( -0.9955873536034882676, 0.000000000000000000, -0.09383933793885600172 ) ) ;
#2290=VERTEX_POINT ( 'NONE', #2095 ) ;
#2292=CARTESIAN_POINT ( 'NONE',  ( -379.9227425692766360, 2.222614453595299867E-15, 174.5211340242017855 ) ) ;
#2293=CARTESIAN_POINT ( 'NONE',  ( -156.9923520473274721, -24.99999999999981881, 556.8176423728723421 ) ) ;
#2294=PLANE ( 'NONE',  #36 ) ;
#2296=AXIS2_PLACEMENT_3D ( 'NONE', #1306, #2986, #4660 ) ;
#2298=AXIS2_PLACEMENT_3D ( 'NONE', #3215, #262, #3620 ) ;
#2299=DIRECTION ( 'NONE',  ( 0.09383933793885568253, -2.673190762809473730E-31, -0.9955873536034882676 ) ) ;
#2300=CARTESIAN_POINT ( 'NONE',  ( -72.60637664584184847, 3.252606517456513302E-16, 552.9197695054128872 ) ) ;
#2301=PRODUCT_CONTEXT ( 'NONE', #632, 'mechanical' ) ;
#2302=CARTESIAN_POINT ( 'NONE',  ( -342.0244061588616091, 3.740497495074990297E-15, 297.0039604601894894 ) ) ;
#2303=CIRCLE ( 'NONE', #634, 31.50000000000114397 ) ;
#2306=CARTESIAN_POINT ( 'NONE',  ( -339.2542556961734590, 25.00000000000018474, 239.6247169981589309 ) ) ;
#2307=ORIENTED_EDGE ( 'NONE', *, *, #4298, .T. ) ;
#2308=ADVANCED_FACE ( 'NONE', ( #1241 ), #2121, .T. ) ;
#2309=DIRECTION ( 'NONE',  ( -1.219242865862094703E-16, 1.000000000000000000, -1.149200448409289593E-17 ) ) ;
#2310=AXIS2_PLACEMENT_3D ( 'NONE', #1079, #2436, #2023 ) ;
#2311=( NAMED_UNIT ( * ) PLANE_ANGLE_UNIT ( ) SI_UNIT ( $, .RADIAN. ) );
#2313=ORIENTED_EDGE ( 'NONE', *, *, #1266, .F. ) ;
#2314=PRODUCT_DEFINITION_CONTEXT ( 'detailed design', #4845, 'design' ) ;
#2315=TOROIDAL_SURFACE ( 'NONE', #1974, 30.50000000000110845, 1.000000000000000000 ) ;
#2317=DIRECTION ( 'NONE',  ( -0.09383933793885568253, 2.673190762809473730E-31, 0.9955873536034882676 ) ) ;
#2319=CARTESIAN_POINT ( 'NONE',  ( -338.5986743560152377, 2.276824562219559311E-15, 39.80450035817695209 ) ) ;
#2323=AXIS2_PLACEMENT_3D ( 'NONE', #5148, #1848, #121 ) ;
#2324=ORIENTED_EDGE ( 'NONE', *, *, #335, .T. ) ;
#2327=CARTESIAN_POINT ( 'NONE',  ( 36.35777514575885760, 2.222614453595284090E-15, 354.7349908125909792 ) ) ;
#2330=DIRECTION ( 'NONE',  ( -1.000000000000000000, -1.219242865862094703E-16, 0.000000000000000000 ) ) ;
#2331=CARTESIAN_POINT ( 'NONE',  ( 36.35777514575907787, 25.00000000000018474, 354.7349908125917750 ) ) ;
#2333=CARTESIAN_POINT ( 'NONE',  ( -12.39202333278750601, -25.00000000000000355, 98.84296066633362443 ) ) ;
#2334=SHAPE_REPRESENTATION ( 'Induction Power Cable Socket', ( #2926 ), #5309 ) ;
#2335=ORIENTED_EDGE ( 'NONE', *, *, #2518, .F. ) ;
#2336=CARTESIAN_POINT ( 'NONE',  ( 4.992201166475765284, 25.00000000000018474, 252.6216919286950429 ) ) ;
#2338=CARTESIAN_POINT ( 'NONE',  ( -328.0684036055322963, 2.759321206427281912E-15, 40.79703369235946298 ) ) ;
#2341=EDGE_CURVE ( 'NONE', #2087, #1199, #4934, .T. ) ;
#2342=EDGE_CURVE ( 'NONE', #3680, #3541, #4673, .T. ) ;
#2343=ORIENTED_EDGE ( 'NONE', *, *, #961, .F. ) ;
#2346=DIRECTION ( 'NONE',  ( -0.09383933793885537722, 2.611561004589082621E-31, 0.9955873536034883786 ) ) ;
#2351=ORIENTED_EDGE ( 'NONE', *, *, #3893, .T. ) ;
#2355=CARTESIAN_POINT ( 'NONE',  ( -72.60637664584184847, 3.252606517456513302E-16, 552.9197695054128872 ) ) ;
#2360=ADVANCED_FACE ( 'NONE', ( #4192, #858 ), #445, .T. ) ;
#2361=CARTESIAN_POINT ( 'NONE',  ( 10.82492224058160879, 25.00000000000018474, 312.2165827548579387 ) ) ;
#2362=CARTESIAN_POINT ( 'NONE',  ( -285.5643670724624599, -25.00000000000003197, 494.2304181244473966 ) ) ;
#2363=CARTESIAN_POINT ( 'NONE',  ( 33.59898979596731294, 5.421010862427522170E-17, 384.0431050523496310 ) ) ;
#2364=TOROIDAL_SURFACE ( 'NONE', #5429, 28.50000000000115463, 1.000000000000000000 ) ;
#2366=CARTESIAN_POINT ( 'NONE',  ( -367.0460729392618191, 25.00000000000018474, 268.0688838304706678 ) ) ;
#2369=LINE ( 'NONE', #4458, #2407 ) ;
#2371=ORIENTED_EDGE ( 'NONE', *, *, #5089, .T. ) ;
#2372=UNCERTAINTY_MEASURE_WITH_UNIT (LENGTH_MEASURE( 1.000000000000000082E-05 ), #4402, 'distance_accuracy_value', 'NONE');
#2374=ORIENTED_EDGE ( 'NONE', *, *, #971, .F. ) ;
#2375=LINE ( 'NONE', #1879, #566 ) ;
#2377=CARTESIAN_POINT ( 'NONE',  ( -361.0769802293077646, 2.222614453595279751E-15, 36.68136974599871536 ) ) ;
#2378=DIRECTION ( 'NONE',  ( 0.09383933793885537722, -2.626968444144180508E-31, -0.9955873536034883786 ) ) ;
#2379=DIRECTION ( 'NONE',  ( 0.9955873536034882676, -5.498835694391114214E-31, 0.09383933793885514130 ) ) ;
#2381=DIRECTION ( 'NONE',  ( -0.01527226085271972227, -2.080004339938201146E-31, -0.9998833722232041143 ) ) ;
#2383=CARTESIAN_POINT ( 'NONE',  ( -57.28677601057280100, 3.252606517456513302E-16, 546.4981013186296650 ) ) ;
#2387=FACE_OUTER_BOUND ( 'NONE', #4633, .T. ) ;
#2388=CARTESIAN_POINT ( 'NONE',  ( -223.9642223310802649, 24.99999999999997158, 534.3227077390027944 ) ) ;
#2389=CARTESIAN_POINT ( 'NONE',  ( -72.60637664584220374, -24.99999999999981881, 552.9197695054134556 ) ) ;
#2392=ORIENTED_EDGE ( 'NONE', *, *, #1203, .F. ) ;
#2393=CARTESIAN_POINT ( 'NONE',  ( 0.07030049710132768581, 1.843143693225357538E-15, 219.5055207296747710 ) ) ;
#2395=CIRCLE ( 'NONE', #19, 27.50000000000126832 ) ;
#2396=DIRECTION ( 'NONE',  ( -0.9955873536034882676, 5.502656983963203831E-31, -0.09383933793885550212 ) ) ;
#2399=EDGE_LOOP ( 'NONE', ( #1991, #3888 ) ) ;
#2404=DIRECTION ( 'NONE',  ( 0.09383933793885568253, -2.673190762809473730E-31, -0.9955873536034882676 ) ) ;
#2405=DIRECTION ( 'NONE',  ( 0.09383933793885537722, -2.626968444144180508E-31, -0.9955873536034883786 ) ) ;
#2407=VECTOR ( 'NONE', #4049, 1000.000000000000114 ) ;
#2409=FACE_OUTER_BOUND ( 'NONE', #2805, .T. ) ;
#2413=VECTOR ( 'NONE', #3248, 1000.000000000000114 ) ;
#2414=DIRECTION ( 'NONE',  ( 0.9955873536034882676, -5.475514420260265162E-31, 0.09383933793885552987 ) ) ;
#2416=VECTOR ( 'NONE', #4308, 1000.000000000000000 ) ;
#2420=AXIS2_PLACEMENT_3D ( 'NONE', #5320, #4498, #1583 ) ;
#2423=CARTESIAN_POINT ( 'NONE',  ( -342.0170653153610374, 25.00000000000018474, 268.9367132353194734 ) ) ;
#2424=CARTESIAN_POINT ( 'NONE',  ( -320.6447527397745034, -25.00000000000003197, 453.8399743637903612 ) ) ;
#2426=CARTESIAN_POINT ( 'NONE',  ( 9.699276322990584731, 1.572093150103981429E-15, 297.8714164406039799 ) ) ;
#2431=ORIENTED_EDGE ( 'NONE', *, *, #78, .F. ) ;
#2432=DIRECTION ( 'NONE',  ( 0.9955873536034882676, -5.498529991225536465E-31, 0.09383933793885551600 ) ) ;
#2433=CARTESIAN_POINT ( 'NONE',  ( -345.9181427152443007, 2.222614453595284090E-15, 117.4603139392499429 ) ) ;
#2434=CARTESIAN_POINT ( 'NONE',  ( -330.4329412795323719, 2.816687638039060658E-15, 198.2700196465188753 ) ) ;
#2436=DIRECTION ( 'NONE',  ( 0.09383933793885568253, -2.673190762809473730E-31, -0.9955873536034882676 ) ) ;
#2437=( BOUNDED_SURFACE ( )  B_SPLINE_SURFACE ( 3, 3, ( 
 ( #2229, #1919, #4015, #3110, #576, #1457, #4781, #3935, #3606, #4395, #1041, #1479, #3958, #1017, #2716, #2664, #987, #3906, #216, #137, #3140, #2300, #4857, #5214, #5160, #2694, #598, #4422, #5264, #3985, #547, #1500, #3081, #4751, #5182, #1063, #4347, #164 ),
 ( #3167, #1094, #2739, #655, #186, #3581, #4371, #1836, #2331, #245, #3551, #3526, #5238, #1424, #2278, #3197, #4826, #1863, #2005, #790, #4126, #2826, #383, #763, #271, #5352, #2450, #3664, #2388, #2886, #4040, #5294, #3686, #4539, #703, #5406, #4939, #356 ),
 ( #1640, #4154, #4071, #3252, #4565, #2773, #2361, #1981, #2034, #4971, #3311, #4449, #4104, #304, #4502, #3225, #1149, #4478, #1618, #2060, #1179, #1948, #2799, #1537, #3634, #2863, #5323, #1587, #1564, #4884, #1122, #3335, #4909, #737, #3709, #1209, #2423, #332 ),
 ( #2474, #3278, #4991, #5379, #3743, #678, #3818, #5012, #1312, #2613, #49, #3357, #1255, #2170, #2108, #3781, #2197, #819, #411, #5070, #2939, #517, #17, #2141, #3764, #4640, #1719, #5096, #2992, #1338, #3870, #932, #4614, #2503, #5043, #1661, #4665, #2084 ),
 ( #848, #3414, #900, #2580, #3025, #4232, #2906, #4587, #2527, #4263, #3440, #4183, #4286, #100, #1686, #4206, #494, #3386, #433, #1778, #3844, #76, #1748, #871, #1282, #4699, #2963, #2551, #4612, #3470, #457, #1232, #1452, #240, #594, #1809, #4726, #3522 ),
 ( #3103, #210, #1831, #5155, #2272, #3952, #3134, #1475, #2689, #1373, #3054, #134, #181, #1890, #955, #2731, #4821, #3932, #1399, #1856, #157, #4748, #4414, #5208, #3543, #2293, #4774, #5179, #4800, #3497, #3077, #2636, #1037, #4314, #2712, #4390, #1914, #614 ),
 ( #572, #981, #5234, #542, #2224, #4367, #3977, #2659, #2327, #3576, #3163, #1419, #1057, #3901, #649, #5130, #4011, #4339, #1014, #2252, #2383, #2355, #2028, #3705, #2823, #673, #2856, #3626, #4880, #1201, #326, #4065, #4497, #1610, #4932, #3659, #2882, #1582 ) ),
 .UNSPECIFIED., .T., .F., .T. ) 
 B_SPLINE_SURFACE_WITH_KNOTS ( ( 4, 3, 4 ),
 ( 4, 2, 2, 2, 2, 2, 2, 2, 2, 2, 2, 2, 2, 2, 2, 2, 2, 2, 4 ),
 ( 0.000000000000000000, 0.5000000000000000000, 1.000000000000000000 ),
 ( 0.000000000000000000, 0.1028767157186024211, 0.2057534314372048423, 0.2571917892965060459, 0.3086301471558072773, 0.3600685050151084532, 0.4115068628744096846, 0.4558387458985032614, 0.4780046874105500776, 0.5001706289225968938, 0.5231687412733679876, 0.5461668536241390814, 0.5921630783256812691, 0.6381593030272234568, 0.6841555277287657555, 0.7631166457965743444, 0.8420777638643828222, 0.9210388819321914111, 1.000000000000000000 ),
 .UNSPECIFIED. ) 
 GEOMETRIC_REPRESENTATION_ITEM ( )  RATIONAL_B_SPLINE_SURFACE ( (
 ( 1.000000000000000000, 1.000000000000000000, 1.000000000000000000, 1.000000000000000000, 1.000000000000000000, 1.000000000000000000, 1.000000000000000000, 1.000000000000000000, 1.000000000000000000, 1.000000000000000000, 1.000000000000000000, 1.000000000000000000, 1.000000000000000000, 1.000000000000000000, 1.000000000000000000, 1.000000000000000000, 1.000000000000000000, 1.000000000000000000, 1.000000000000000000, 1.000000000000000000, 1.000000000000000000, 1.000000000000000000, 1.000000000000000000, 1.000000000000000000, 1.000000000000000000, 1.000000000000000000, 1.000000000000000000, 1.000000000000000000, 1.000000000000000000, 1.000000000000000000, 1.000000000000000000, 1.000000000000000000, 1.000000000000000000, 1.000000000000000000, 1.000000000000000000, 1.000000000000000000, 1.000000000000000000, 1.000000000000000000),
 ( 0.3333333333333333703, 0.3333333333333333703, 0.3333333333333333703, 0.3333333333333333703, 0.3333333333333333703, 0.3333333333333333703, 0.3333333333333333703, 0.3333333333333333703, 0.3333333333333333703, 0.3333333333333333703, 0.3333333333333333703, 0.3333333333333333703, 0.3333333333333333703, 0.3333333333333333703, 0.3333333333333333703, 0.3333333333333333703, 0.3333333333333333703, 0.3333333333333333703, 0.3333333333333333703, 0.3333333333333333703, 0.3333333333333333703, 0.3333333333333333703, 0.3333333333333333703, 0.3333333333333333703, 0.3333333333333333703, 0.3333333333333333703, 0.3333333333333333703, 0.3333333333333333703, 0.3333333333333333703, 0.3333333333333333703, 0.3333333333333333703, 0.3333333333333333703, 0.3333333333333333703, 0.3333333333333333703, 0.3333333333333333703, 0.3333333333333333703, 0.3333333333333333703, 0.3333333333333333703),
 ( 0.3333333333333333703, 0.3333333333333333703, 0.3333333333333333703, 0.3333333333333333703, 0.3333333333333333703, 0.3333333333333333703, 0.3333333333333333703, 0.3333333333333333703, 0.3333333333333333703, 0.3333333333333333703, 0.3333333333333333703, 0.3333333333333333703, 0.3333333333333333703, 0.3333333333333333703, 0.3333333333333333703, 0.3333333333333333703, 0.3333333333333333703, 0.3333333333333333703, 0.3333333333333333703, 0.3333333333333333703, 0.3333333333333333703, 0.3333333333333333703, 0.3333333333333333703, 0.3333333333333333703, 0.3333333333333333703, 0.3333333333333333703, 0.3333333333333333703, 0.3333333333333333703, 0.3333333333333333703, 0.3333333333333333703, 0.3333333333333333703, 0.3333333333333333703, 0.3333333333333333703, 0.3333333333333333703, 0.3333333333333333703, 0.3333333333333333703, 0.3333333333333333703, 0.3333333333333333703),
 ( 1.000000000000000000, 1.000000000000000000, 1.000000000000000000, 1.000000000000000000, 1.000000000000000000, 1.000000000000000000, 1.000000000000000000, 1.000000000000000000, 1.000000000000000000, 1.000000000000000000, 1.000000000000000000, 1.000000000000000000, 1.000000000000000000, 1.000000000000000000, 1.000000000000000000, 1.000000000000000000, 1.000000000000000000, 1.000000000000000000, 1.000000000000000000, 1.000000000000000000, 1.000000000000000000, 1.000000000000000000, 1.000000000000000000, 1.000000000000000000, 1.000000000000000000, 1.000000000000000000, 1.000000000000000000, 1.000000000000000000, 1.000000000000000000, 1.000000000000000000, 1.000000000000000000, 1.000000000000000000, 1.000000000000000000, 1.000000000000000000, 1.000000000000000000, 1.000000000000000000, 1.000000000000000000, 1.000000000000000000),
 ( 0.3333333333333333703, 0.3333333333333333703, 0.3333333333333333703, 0.3333333333333333703, 0.3333333333333333703, 0.3333333333333333703, 0.3333333333333333703, 0.3333333333333333703, 0.3333333333333333703, 0.3333333333333333703, 0.3333333333333333703, 0.3333333333333333703, 0.3333333333333333703, 0.3333333333333333703, 0.3333333333333333703, 0.3333333333333333703, 0.3333333333333333703, 0.3333333333333333703, 0.3333333333333333703, 0.3333333333333333703, 0.3333333333333333703, 0.3333333333333333703, 0.3333333333333333703, 0.3333333333333333703, 0.3333333333333333703, 0.3333333333333333703, 0.3333333333333333703, 0.3333333333333333703, 0.3333333333333333703, 0.3333333333333333703, 0.3333333333333333703, 0.3333333333333333703, 0.3333333333333333703, 0.3333333333333333703, 0.3333333333333333703, 0.3333333333333333703, 0.3333333333333333703, 0.3333333333333333703),
 ( 0.3333333333333333703, 0.3333333333333333703, 0.3333333333333333703, 0.3333333333333333703, 0.3333333333333333703, 0.3333333333333333703, 0.3333333333333333703, 0.3333333333333333703, 0.3333333333333333703, 0.3333333333333333703, 0.3333333333333333703, 0.3333333333333333703, 0.3333333333333333703, 0.3333333333333333703, 0.3333333333333333703, 0.3333333333333333703, 0.3333333333333333703, 0.3333333333333333703, 0.3333333333333333703, 0.3333333333333333703, 0.3333333333333333703, 0.3333333333333333703, 0.3333333333333333703, 0.3333333333333333703, 0.3333333333333333703, 0.3333333333333333703, 0.3333333333333333703, 0.3333333333333333703, 0.3333333333333333703, 0.3333333333333333703, 0.3333333333333333703, 0.3333333333333333703, 0.3333333333333333703, 0.3333333333333333703, 0.3333333333333333703, 0.3333333333333333703, 0.3333333333333333703, 0.3333333333333333703),
 ( 1.000000000000000000, 1.000000000000000000, 1.000000000000000000, 1.000000000000000000, 1.000000000000000000, 1.000000000000000000, 1.000000000000000000, 1.000000000000000000, 1.000000000000000000, 1.000000000000000000, 1.000000000000000000, 1.000000000000000000, 1.000000000000000000, 1.000000000000000000, 1.000000000000000000, 1.000000000000000000, 1.000000000000000000, 1.000000000000000000, 1.000000000000000000, 1.000000000000000000, 1.000000000000000000, 1.000000000000000000, 1.000000000000000000, 1.000000000000000000, 1.000000000000000000, 1.000000000000000000, 1.000000000000000000, 1.000000000000000000, 1.000000000000000000, 1.000000000000000000, 1.000000000000000000, 1.000000000000000000, 1.000000000000000000, 1.000000000000000000, 1.000000000000000000, 1.000000000000000000, 1.000000000000000000, 1.000000000000000000) ) ) 
 REPRESENTATION_ITEM ( '' )  SURFACE ( )  );
#2441=ORIENTED_EDGE ( 'NONE', *, *, #2578, .F. ) ;
#2442=DIRECTION ( 'NONE',  ( 0.09383933793885568253, -2.673190762809473730E-31, -0.9955873536034882676 ) ) ;
#2443=AXIS2_PLACEMENT_3D ( 'NONE', #5206, #3899, #613 ) ;
#2444=CARTESIAN_POINT ( 'NONE',  ( -346.1058213911226176, 0.000000000000000000, 119.4514886464559424 ) ) ;
#2447=CIRCLE ( 'NONE', #1912, 31.50000000000114397 ) ;
#2450=CARTESIAN_POINT ( 'NONE',  ( -174.3534642324312358, 25.00000000000018474, 552.7876087698487027 ) ) ;
#2451=CARTESIAN_POINT ( 'NONE',  ( -207.8397519515722252, -25.00000000000003197, 541.5412455041529256 ) ) ;
#2452=EDGE_CURVE ( 'NONE', #4297, #1438, #1794, .T. ) ;
#2454=CARTESIAN_POINT ( 'NONE',  ( -39.32426838448843398, 3.740497495074990297E-15, 499.4571537926191240 ) ) ;
#2455=ORIENTED_EDGE ( 'NONE', *, *, #1403, .F. ) ;
#2456=CARTESIAN_POINT ( 'NONE',  ( -0.6802310551622114954, 2.222614453595284090E-15, 47.14310755735262859 ) ) ;
#2457=EDGE_CURVE ( 'NONE', #281, #4617, #4328, .T. ) ;
#2459=EDGE_LOOP ( 'NONE', ( #4020, #1573 ) ) ;
#2460=PRODUCT ( 'Induction Power Cable Socket', 'Induction Power Cable Socket', '', ( #2301 ) ) ;
#2461=FACE_OUTER_BOUND ( 'NONE', #714, .T. ) ;
#2465=DIRECTION ( 'NONE',  ( 1.000000000000000000, -5.777789833161702304E-31, 0.000000000000000000 ) ) ;
#2466=ORIENTED_EDGE ( 'NONE', *, *, #5358, .T. ) ;
#2467=ORIENTED_EDGE ( 'NONE', *, *, #3329, .T. ) ;
#2468=DIRECTION ( 'NONE',  ( -0.09383933793885568253, 2.673190762809473730E-31, 0.9955873536034882676 ) ) ;
#2469=DIRECTION ( 'NONE',  ( 0.9955873536034882676, -5.502656983963330823E-31, 0.09383933793885547436 ) ) ;
#2474=CARTESIAN_POINT ( 'NONE',  ( -13.17877320795268759, 1.897353801849632760E-15, 47.33401081801291355 ) ) ;
#2475=CARTESIAN_POINT ( 'NONE',  ( -57.28677601057306390, -24.99999999999981881, 546.4981013186294376 ) ) ;
#2477=VERTEX_POINT ( 'NONE', #1760 ) ;
#2479=DIRECTION ( 'NONE',  ( 0.9998833722232041143, -6.779273404243022909E-31, -0.01527226085271993737 ) ) ;
#2481=VECTOR ( 'NONE', #1324, 1000.000000000000114 ) ;
#2489=DIRECTION ( 'NONE',  ( 0.01527226085271972227, 2.095411779493299033E-31, 0.9998833722232041143 ) ) ;
#2496=EDGE_CURVE ( 'NONE', #4831, #3541, #4256, .T. ) ;
#2499=B_SPLINE_CURVE_WITH_KNOTS ( 'NONE', 3,
 ( #2577, #4990, #381, #1231, #4153, #817, #5431, #2502, #3385, #2059, #5042, #4182, #432, #4639, #2139, #3356, #2083, #4262, #5405, #2905, #870, #3334, #1639, #493, #2169, #5011, #2550, #3023, #3843, #3763, #2938, #75, #410, #1253, #4613, #3817, #4664, #2991 ),
 .UNSPECIFIED., .F., .F.,
 ( 4, 2, 2, 2, 2, 2, 2, 2, 2, 2, 2, 2, 2, 2, 2, 2, 2, 2, 4 ),
 ( 0.000000000000000000, 0.1028767157186024211, 0.2057534314372048423, 0.2571917892965060459, 0.3086301471558072773, 0.3600685050151084532, 0.4115068628744096846, 0.4558387458985032614, 0.4780046874105500776, 0.5001706289225968938, 0.5231687412733679876, 0.5461668536241390814, 0.5921630783256812691, 0.6381593030272234568, 0.6841555277287657555, 0.7631166457965743444, 0.8420777638643828222, 0.9210388819321914111, 1.000000000000000000 ),
 .UNSPECIFIED. ) ;
#2500=CIRCLE ( 'NONE', #999, 4.382543221487789964 ) ;
#2502=CARTESIAN_POINT ( 'NONE',  ( 11.65205807320734976, 3.740497495074990297E-15, 340.0738060255405912 ) ) ;
#2503=CARTESIAN_POINT ( 'NONE',  ( -330.1866567701584927, 3.740497495074990297E-15, 374.2973685668102917 ) ) ;
#2504=CYLINDRICAL_SURFACE ( 'NONE', #390, 21.00000000000012790 ) ;
#2505=CIRCLE ( 'NONE', #831, 28.50000000000127898 ) ;
#2506=AXIS2_PLACEMENT_3D ( 'NONE', #2883, #786, #1174 ) ;
#2508=EDGE_LOOP ( 'NONE', ( #139, #972 ) ) ;
#2511=ORIENTED_EDGE ( 'NONE', *, *, #2031, .T. ) ;
#2514=DIRECTION ( 'NONE',  ( -0.9955873536034883786, 5.496925049605202091E-31, -0.09383933793885522456 ) ) ;
#2515=EDGE_CURVE ( 'NONE', #4297, #3915, #2395, .T. ) ;
#2516=CARTESIAN_POINT ( 'NONE',  ( -351.6990976162155107, 2.276824562219559311E-15, 238.4517252739237847 ) ) ;
#2517=CARTESIAN_POINT ( 'NONE',  ( -321.2769280446073026, 3.850615185981194977E-15, 181.0532423161974975 ) ) ;
#2518=EDGE_CURVE ( 'NONE', #2126, #342, #4073, .T. ) ;
#2522=CARTESIAN_POINT ( 'NONE',  ( -0.6802310551622114954, 2.222614453595284090E-15, 47.14310755735262859 ) ) ;
#2523=LINE ( 'NONE', #71, #1335 ) ;
#2524=EDGE_CURVE ( 'NONE', #2290, #229, #4887, .T. ) ;
#2525=CARTESIAN_POINT ( 'NONE',  ( -344.4167133082243595, 2.222614453595284090E-15, 101.5309162815936048 ) ) ;
#2527=CARTESIAN_POINT ( 'NONE',  ( 11.35554381054933160, -24.99999999999981881, 353.5846600851155017 ) ) ;
#2529=AXIS2_PLACEMENT_3D ( 'NONE', #2538, #1193, #3698 ) ;
#2532=DIRECTION ( 'NONE',  ( 0.09383933793885568253, -2.673190762809473730E-31, -0.9955873536034882676 ) ) ;
#2536=LINE ( 'NONE', #1731, #1073 ) ;
#2538=CARTESIAN_POINT ( 'NONE',  ( -346.0119820531830328, 0.000000000000000000, 118.4559012928528858 ) ) ;
#2542=ORIENTED_EDGE ( 'NONE', *, *, #2274, .F. ) ;
#2543=EDGE_LOOP ( 'NONE', ( #946, #4998 ) ) ;
#2544=ORIENTED_EDGE ( 'NONE', *, *, #1787, .T. ) ;
#2550=CARTESIAN_POINT ( 'NONE',  ( -167.9289969670494997, 3.740497495074990297E-15, 528.5729890193238134 ) ) ;
#2551=CARTESIAN_POINT ( 'NONE',  ( -198.3455225866221667, -25.00000000000003197, 518.3576047634796851 ) ) ;
#2552=CARTESIAN_POINT ( 'NONE',  ( -364.1439395362591540, 2.222614453595284090E-15, 237.2787335496894343 ) ) ;
#2554=VERTEX_POINT ( 'NONE', #5109 ) ;
#2556=DIRECTION ( 'NONE',  ( -0.9955873536034882676, 5.452307672560245432E-31, -0.09383933793885568253 ) ) ;
#2559=CARTESIAN_POINT ( 'NONE',  ( -323.7051989975983588, 2.222614453595284090E-15, 41.20828864675230108 ) ) ;
#2560=PLANE ( 'NONE',  #5376 ) ;
#2561=CARTESIAN_POINT ( 'NONE',  ( -86.97194166595193110, -24.99999999999981881, 531.0655262460722952 ) ) ;
#2564=CARTESIAN_POINT ( 'NONE',  ( -353.5191290882918338, 0.000000000000000000, 198.1028895811327573 ) ) ;
#2565=AXIS2_PLACEMENT_3D ( 'NONE', #2000, #4474, #2414 ) ;
#2568=AXIS2_PLACEMENT_3D ( 'NONE', #1139, #2845, #2814 ) ;
#2571=CARTESIAN_POINT ( 'NONE',  ( -311.1905691331858179, 2.276824562219544323E-15, 41.38342604719807127 ) ) ;
#2574=AXIS2_PLACEMENT_3D ( 'NONE', #690, #1049, #2432 ) ;
#2576=CIRCLE ( 'NONE', #2053, 12.50000000000003197 ) ;
#2577=CARTESIAN_POINT ( 'NONE',  ( -13.17877320795226659, 1.897353801849669836E-15, 47.33401081801162746 ) ) ;
#2578=EDGE_CURVE ( 'NONE', #3236, #3490, #2536, .T. ) ;
#2580=CARTESIAN_POINT ( 'NONE',  ( 0.07030049708446614587, -25.00000000000000355, 219.5055207296742026 ) ) ;
#2581=CARTESIAN_POINT ( 'NONE',  ( -344.1351952944073105, 5.421010862427522170E-17, 98.54415422078299969 ) ) ;
#2583=EDGE_CURVE ( 'NONE', #2126, #4277, #1511, .T. ) ;
#2589=CARTESIAN_POINT ( 'NONE',  ( -0.8482259245422840710, 2.276824562219559311E-15, 36.14439046289818691 ) ) ;
#2591=FACE_OUTER_BOUND ( 'NONE', #2459, .T. ) ;
#2592=CIRCLE ( 'NONE', #5390, 1.000000000000000888 ) ;
#2593=ORIENTED_EDGE ( 'NONE', *, *, #85, .T. ) ;
#2598=CARTESIAN_POINT ( 'NONE',  ( -167.9289969670494997, 3.740497495074990297E-15, 528.5729890193238134 ) ) ;
#2599=CARTESIAN_POINT ( 'NONE',  ( -19.78983854945498422, 2.222614453595284090E-15, 515.1268587725810448 ) ) ;
#2601=ADVANCED_FACE ( 'NONE', ( #967 ), #2560, .T. ) ;
#2605=ORIENTED_EDGE ( 'NONE', *, *, #3499, .F. ) ;
#2606=CARTESIAN_POINT ( 'NONE',  ( -348.7799179161582970, 14.95948628165116823, 101.1196613272007738 ) ) ;
#2608=ADVANCED_FACE ( 'NONE', ( #915 ), #1268, .T. ) ;
#2610=FACE_OUTER_BOUND ( 'NONE', #3732, .T. ) ;
#2611=ORIENTED_EDGE ( 'NONE', *, *, #823, .F. ) ;
#2613=CARTESIAN_POINT ( 'NONE',  ( 8.821273309647297722, 3.740497495074990297E-15, 380.5076279642372015 ) ) ;
#2618=ORIENTED_EDGE ( 'NONE', *, *, #983, .T. ) ;
#2621=ORIENTED_EDGE ( 'NONE', *, *, #2200, .F. ) ;
#2622=CARTESIAN_POINT ( 'NONE',  ( -57.28677601057280100, 3.252606517456513302E-16, 546.4981013186296650 ) ) ;
#2624=CARTESIAN_POINT ( 'NONE',  ( -330.1866567701584927, 3.740497495074990297E-15, 374.2973685668102917 ) ) ;
#2625=CARTESIAN_POINT ( 'NONE',  ( -264.1404626571534777, 2.222614453595284090E-15, 511.7445549721628595 ) ) ;
#2626=DIRECTION ( 'NONE',  ( -0.9998833722232041143, 6.892903270961872452E-31, 0.01527226085271972227 ) ) ;
#2631=DIRECTION ( 'NONE',  ( 0.09383933793885568253, -2.673190762809473730E-31, -0.9955873536034882676 ) ) ;
#2634=EDGE_LOOP ( 'NONE', ( #2232, #2657, #1711, #2335 ) ) ;
#2635=DIRECTION ( 'NONE',  ( 1.000000000000000000, -3.851859888774468203E-31, 0.000000000000000000 ) ) ;
#2636=CARTESIAN_POINT ( 'NONE',  ( -320.6447527397745034, -25.00000000000003197, 453.8399743637903612 ) ) ;
#2637=CARTESIAN_POINT ( 'NONE',  ( -365.8191009029663974, 5.636683259291067391E-15, 36.23439996194949941 ) ) ;
#2638=ORIENTED_EDGE ( 'NONE', *, *, #765, .F. ) ;
#2639=DIRECTION ( 'NONE',  ( 0.9998833722232040033, -6.797399803719615819E-31, -0.01527226085271964420 ) ) ;
#2641=CARTESIAN_POINT ( 'NONE',  ( 35.78913469918423829, 0.000000000000000000, 310.6402212931345161 ) ) ;
#2643=DIRECTION ( 'NONE',  ( -0.9955873536034882676, 5.453577263127812432E-31, -0.09383933793885552987 ) ) ;
#2644=CARTESIAN_POINT ( 'NONE',  ( -342.0170653153606395, 3.740497495074990297E-15, 268.9367132353195302 ) ) ;
#2645=CARTESIAN_POINT ( 'NONE',  ( 18.31346110193232590, 2.222614453595284090E-15, 444.2932575970293101 ) ) ;
#2647=EDGE_CURVE ( 'NONE', #4331, #4307, #4244, .T. ) ;
#2648=EDGE_CURVE ( 'NONE', #3875, #2651, #549, .T. ) ;
#2651=VERTEX_POINT ( 'NONE', #2118 ) ;
#2653=DIRECTION ( 'NONE',  ( -5.679099018122554920E-31, -1.000000000000000000, 2.149753974990777610E-31 ) ) ;
#2654=DIRECTION ( 'NONE',  ( -0.9955873536034882676, 5.502656983963321189E-31, -0.09383933793885573804 ) ) ;
#2657=ORIENTED_EDGE ( 'NONE', *, *, #4855, .T. ) ;
#2659=CARTESIAN_POINT ( 'NONE',  ( 36.66581985038869362, 3.252606517456513302E-16, 340.1662229844753256 ) ) ;
#2660=CARTESIAN_POINT ( 'NONE',  ( -338.5048350180761076, 2.276824562219559311E-15, 38.80891300457378890 ) ) ;
#2662=AXIS2_PLACEMENT_3D ( 'NONE', #4949, #3315, #745 ) ;
#2663=ORIENTED_EDGE ( 'NONE', *, *, #335, .F. ) ;
#2664=CARTESIAN_POINT ( 'NONE',  ( -14.89480152442229688, 0.000000000000000000, 508.6517828409968729 ) ) ;
#2669=CARTESIAN_POINT ( 'NONE',  ( -364.1439395362591540, 2.222614453595284090E-15, 237.2787335496894343 ) ) ;
#2672=AXIS2_PLACEMENT_3D ( 'NONE', #4700, #101, #1779 ) ;
#2674=CIRCLE ( 'NONE', #3997, 4.382543221487789964 ) ;
#2675=CARTESIAN_POINT ( 'NONE',  ( -349.8593949086763928, 2.222614453595284090E-15, 159.2749827905956010 ) ) ;
#2676=FACE_OUTER_BOUND ( 'NONE', #3589, .T. ) ;
#2678=ORIENTED_EDGE ( 'NONE', *, *, #2208, .T. ) ;
#2681=DIRECTION ( 'NONE',  ( 0.09383933793885568253, -2.673190762809473730E-31, -0.9955873536034882676 ) ) ;
#2683=CARTESIAN_POINT ( 'NONE',  ( -345.9181427152443007, 2.222614453595284090E-15, 117.4603139392499429 ) ) ;
#2689=CARTESIAN_POINT ( 'NONE',  ( 36.35777514575907787, -24.99999999999981881, 354.7349908125917750 ) ) ;
#2690=DIRECTION ( 'NONE',  ( 0.9955873536034882676, 0.000000000000000000, 0.09383933793885600172 ) ) ;
#2692=CIRCLE ( 'NONE', #3929, 22.67218956682437536 ) ;
#2694=CARTESIAN_POINT ( 'NONE',  ( -156.9923520473269321, 0.000000000000000000, 556.8176423728721147 ) ) ;
#2695=VERTEX_POINT ( 'NONE', #553 ) ;
#2696=CARTESIAN_POINT ( 'NONE',  ( 31.14585677005056041, 25.00000000000018474, 398.7793066466517757 ) ) ;
#2705=CARTESIAN_POINT ( 'NONE',  ( -311.1905691331858179, 2.276824562219544323E-15, 41.38342604719806417 ) ) ;
#2707=DIRECTION ( 'NONE',  ( -5.679099018122554920E-31, -1.000000000000000000, 2.149753974990777610E-31 ) ) ;
#2708=CARTESIAN_POINT ( 'NONE',  ( -13.17877320795226659, 1.897353801849669836E-15, 47.33401081801162746 ) ) ;
#2709=CARTESIAN_POINT ( 'NONE',  ( -342.9618789639491752, 2.813531315051557923E-15, 39.39324540378412109 ) ) ;
#2712=CARTESIAN_POINT ( 'NONE',  ( -360.7307227603797060, -24.99999999999981881, 354.4373729494859049 ) ) ;
#2713=DIRECTION ( 'NONE',  ( 0.09383933793885568253, -2.673190762809473730E-31, -0.9955873536034882676 ) ) ;
#2715=DIRECTION ( 'NONE',  ( -0.9955873536034883786, 5.430490990731020552E-31, -0.09383933793885548824 ) ) ;
#2716=CARTESIAN_POINT ( 'NONE',  ( -1.533280346156490337, 2.222614453595284090E-15, 488.4857301958385278 ) ) ;
#2717=ORIENTED_EDGE ( 'NONE', *, *, #894, .T. ) ;
#2718=CARTESIAN_POINT ( 'NONE',  ( -122.4270646331732451, 25.00000000000018474, 560.5113017241552598 ) ) ;
#2719=ORIENTED_EDGE ( 'NONE', *, *, #560, .F. ) ;
#2721=DIRECTION ( 'NONE',  ( -1.000000000000000000, -1.219242865862094703E-16, 0.000000000000000000 ) ) ;
#2722=VERTEX_POINT ( 'NONE', #2338 ) ;
#2724=CARTESIAN_POINT ( 'NONE',  ( -351.7361816674535362, 5.421010862427522170E-17, 179.1867298626658283 ) ) ;
#2728=EDGE_LOOP ( 'NONE', ( #2955, #3125 ) ) ;
#2730=CARTESIAN_POINT ( 'NONE',  ( -359.3101886666408404, 0.000000000000000000, 100.1271279930180356 ) ) ;
#2731=CARTESIAN_POINT ( 'NONE',  ( -14.89480152442222582, -24.99999999999981881, 508.6517828409982940 ) ) ;
#2733=TOROIDAL_SURFACE ( 'NONE', #4585, 30.50000000000110845, 1.000000000000000000 ) ;
#2738=CARTESIAN_POINT ( 'NONE',  ( -323.1742634138752805, 5.712857831165392007E-15, 179.8699762867167351 ) ) ;
#2739=CARTESIAN_POINT ( 'NONE',  ( 16.26935751051938439, 25.00000000000000355, 140.3055424402287770 ) ) ;
#2741=CARTESIAN_POINT ( 'NONE',  ( -299.8611223228771792, -25.00000000000003197, 439.6443911606498887 ) ) ;
#2744=VECTOR ( 'NONE', #306, 1000.000000000000114 ) ;
#2746=CARTESIAN_POINT ( 'NONE',  ( -16.96312831416361533, 25.00000000000018474, 463.2830513152442222 ) ) ;
#2750=CIRCLE ( 'NONE', #3124, 21.00000000000012790 ) ;
#2755=AXIS2_PLACEMENT_3D ( 'NONE', #2581, #1339, #4992 ) ;
#2762=AXIS2_PLACEMENT_3D ( 'NONE', #2433, #3619, #717 ) ;
#2765=EDGE_CURVE ( 'NONE', #689, #4644, #5194, .T. ) ;
#2769=PLANE ( 'NONE',  #1267 ) ;
#2772=CARTESIAN_POINT ( 'NONE',  ( 11.81831109762776322, 2.276824562219553001E-15, 46.95220429669362971 ) ) ;
#2773=CARTESIAN_POINT ( 'NONE',  ( 9.699276322990401766, 25.00000000000018474, 297.8714164406044915 ) ) ;
#2775=CARTESIAN_POINT ( 'NONE',  ( -1.533280346156948193, -24.99999999999981881, 488.4857301958397784 ) ) ;
#2779=CARTESIAN_POINT ( 'NONE',  ( -167.9289969670495282, 25.00000000000018474, 528.5729890193230176 ) ) ;
#2782=DIRECTION ( 'NONE',  ( -0.09383933793885536334, 2.626968444144180070E-31, 0.9955873536034882676 ) ) ;
#2784=ORIENTED_EDGE ( 'NONE', *, *, #4460, .F. ) ;
#2785=CIRCLE ( 'NONE', #4547, 4.382543221487789076 ) ;
#2786=ORIENTED_EDGE ( 'NONE', *, *, #4793, .F. ) ;
#2789=CARTESIAN_POINT ( 'NONE',  ( -344.4167133082243595, 2.222614453595284090E-15, 101.5309162815936048 ) ) ;
#2794=DIRECTION ( 'NONE',  ( -0.09383933793885537722, 2.626968444144180508E-31, 0.9955873536034883786 ) ) ;
#2795=DIRECTION ( 'NONE',  ( 0.09383933793885537722, -2.626968444144180508E-31, -0.9955873536034883786 ) ) ;
#2798=CARTESIAN_POINT ( 'NONE',  ( -338.5986743560152377, 2.276824562219559311E-15, 39.80450035817695209 ) ) ;
#2799=CARTESIAN_POINT ( 'NONE',  ( -86.97194166595193110, 25.00000000000018474, 531.0655262460722952 ) ) ;
#2800=CARTESIAN_POINT ( 'NONE',  ( 18.31346110193232590, 2.222614453595284090E-15, 444.2932575970293101 ) ) ;
#2802=CIRCLE ( 'NONE', #1402, 12.50000000000003197 ) ;
#2804=CARTESIAN_POINT ( 'NONE',  ( -334.2906958041451162, 24.99999999999997158, 430.9840019716597226 ) ) ;
#2805=EDGE_LOOP ( 'NONE', ( #2618, #350, #2990, #5165 ) ) ;
#2810=ORIENTED_EDGE ( 'NONE', *, *, #2816, .F. ) ;
#2811=DIRECTION ( 'NONE',  ( 0.01527226085271972227, 2.095411779493299033E-31, 0.9998833722232041143 ) ) ;
#2814=DIRECTION ( 'NONE',  ( -0.9955873536034884896, 5.465719896581968711E-31, -0.09383933793885443353 ) ) ;
#2816=EDGE_CURVE ( 'NONE', #1728, #4985, #4678, .T. ) ;
#2818=EDGE_CURVE ( 'NONE', #5060, #5244, #3558, .T. ) ;
#2819=DIRECTION ( 'NONE',  ( 0.09383933793885568253, -2.673190762809473730E-31, -0.9955873536034882676 ) ) ;
#2820=ORIENTED_EDGE ( 'NONE', *, *, #1266, .T. ) ;
#2823=CARTESIAN_POINT ( 'NONE',  ( -122.4270646331731598, 3.252606517456513302E-16, 560.5113017241549187 ) ) ;
#2824=CARTESIAN_POINT ( 'NONE',  ( -318.3107145942876173, 2.222614453595271862E-15, 160.2397472284629885 ) ) ;
#2826=CARTESIAN_POINT ( 'NONE',  ( -72.60637664584220374, 25.00000000000018474, 552.9197695054134556 ) ) ;
#2828=CARTESIAN_POINT ( 'NONE',  ( -105.2090356704105147, 2.222614453595284090E-15, 560.1816718768288865 ) ) ;
#2829=AXIS2_PLACEMENT_3D ( 'NONE', #4223, #3409, #3015 ) ;
#2831=CARTESIAN_POINT ( 'NONE',  ( -23.53079058812344471, 25.00000000000018474, 476.4235034963351154 ) ) ;
#2833=AXIS2_PLACEMENT_3D ( 'NONE', #4627, #3428, #1671 ) ;
#2836=( NAMED_UNIT ( * ) SI_UNIT ( $, .STERADIAN. ) SOLID_ANGLE_UNIT ( ) );
#2839=ORIENTED_EDGE ( 'NONE', *, *, #2914, .T. ) ;
#2843=DIRECTION ( 'NONE',  ( -0.9955873536034882676, 5.436595176548168253E-31, -0.09383933793885512742 ) ) ;
#2845=DIRECTION ( 'NONE',  ( 0.09383933793885568253, -2.673190762809473730E-31, -0.9955873536034882676 ) ) ;
#2852=EDGE_CURVE ( 'NONE', #5244, #4403, #1682, .T. ) ;
#2856=CARTESIAN_POINT ( 'NONE',  ( -174.3534642324304116, 5.421010862427522170E-17, 552.7876087698471110 ) ) ;
#2857=FACE_BOUND ( 'NONE', #757, .T. ) ;
#2858=VECTOR ( 'NONE', #3758, 1000.000000000000114 ) ;
#2859=CIRCLE ( 'NONE', #4345, 30.50000000000124345 ) ;
#2861=CIRCLE ( 'NONE', #4419, 12.50000000000003197 ) ;
#2862=DIRECTION ( 'NONE',  ( -5.720779902258401340E-31, -1.000000000000000000, 2.099398147291833041E-31 ) ) ;
#2863=CARTESIAN_POINT ( 'NONE',  ( -152.2642418385221674, 25.00000000000018474, 532.1805559224801527 ) ) ;
#2864=CARTESIAN_POINT ( 'NONE',  ( -264.1404626571534777, 2.222614453595284090E-15, 511.7445549721628595 ) ) ;
#2865=ORIENTED_EDGE ( 'NONE', *, *, #2765, .F. ) ;
#2866=CARTESIAN_POINT ( 'NONE',  ( -23.53079058812296154, 3.740497495074990297E-15, 476.4235034963361954 ) ) ;
#2873=CARTESIAN_POINT ( 'NONE',  ( -353.5191290882918338, 0.000000000000000000, 198.1028895811323025 ) ) ;
#2877=VERTEX_POINT ( 'NONE', #279 ) ;
#2881=AXIS2_PLACEMENT_3D ( 'NONE', #5258, #2794, #5318 ) ;
#2882=CARTESIAN_POINT ( 'NONE',  ( -367.0460729392618759, 0.000000000000000000, 268.0688838304710089 ) ) ;
#2883=CARTESIAN_POINT ( 'NONE',  ( -347.8887688119603467, 2.222614453595284090E-15, 138.3676483649222178 ) ) ;
#2886=CARTESIAN_POINT ( 'NONE',  ( -264.1404626571541598, 24.99999999999997158, 511.7445549721641100 ) ) ;
#2887=CARTESIAN_POINT ( 'NONE',  ( 33.59898979596707136, -24.99999999999981881, 384.0431050523492900 ) ) ;
#2888=EDGE_CURVE ( 'NONE', #3915, #4297, #3105, .T. ) ;
#2893=ORIENTED_EDGE ( 'NONE', *, *, #3885, .T. ) ;
#2896=DIRECTION ( 'NONE',  ( 0.09383933793885568253, -2.673190762809473730E-31, -0.9955873536034882676 ) ) ;
#2899=ORIENTED_EDGE ( 'NONE', *, *, #156, .F. ) ;
#2902=CYLINDRICAL_SURFACE ( 'NONE', #3711, 27.50000000000126121 ) ;
#2903=LINE ( 'NONE', #5403, #570 ) ;
#2905=CARTESIAN_POINT ( 'NONE',  ( -63.04765821499436385, 1.843143693225357538E-15, 521.0401840782876661 ) ) ;
#2906=CARTESIAN_POINT ( 'NONE',  ( 10.82492224058160879, -24.99999999999981881, 312.2165827548579387 ) ) ;
#2907=DIRECTION ( 'NONE',  ( 0.9955873536034883786, -5.498529991225532086E-31, 0.09383933793885522456 ) ) ;
#2910=EDGE_CURVE ( 'NONE', #1728, #195, #4476, .T. ) ;
#2911=CIRCLE ( 'NONE', #1775, 30.50000000000124345 ) ;
#2913=LINE ( 'NONE', #4110, #1796 ) ;
#2914=EDGE_CURVE ( 'NONE', #1142, #8, #2303, .T. ) ;
#2917=ORIENTED_EDGE ( 'NONE', *, *, #5425, .F. ) ;
#2918=EDGE_LOOP ( 'NONE', ( #2374, #2371, #1952, #2343 ) ) ;
#2919=DIRECTION ( 'NONE',  ( 0.09383933793885568253, -2.673190762809473730E-31, -0.9955873536034882676 ) ) ;
#2921=DIRECTION ( 'NONE',  ( 0.09383933793885568253, -2.673190762809473730E-31, -0.9955873536034882676 ) ) ;
#2923=DIRECTION ( 'NONE',  ( -0.09383933793885537722, 2.626968444144180508E-31, 0.9955873536034883786 ) ) ;
#2925=AXIS2_PLACEMENT_3D ( 'NONE', #596, #5427, #1683 ) ;
#2926=AXIS2_PLACEMENT_3D ( 'NONE', #4646, #959, #1347 ) ;
#2932=AXIS2_PLACEMENT_3D ( 'NONE', #4033, #3519, #4817 ) ;
#2937=AXIS2_PLACEMENT_3D ( 'NONE', #4010, #325, #1999 ) ;
#2938=CARTESIAN_POINT ( 'NONE',  ( -268.5984117390374877, 3.740497495074990297E-15, 475.6392848759629715 ) ) ;
#2939=CARTESIAN_POINT ( 'NONE',  ( -68.63039925413394826, 1.572093150103981429E-15, 524.1455590405157636 ) ) ;
#2940=CARTESIAN_POINT ( 'NONE',  ( -364.1439395362590972, 2.398458366376004494E-13, 237.2787335496881553 ) ) ;
#2942=AXIS2_PLACEMENT_3D ( 'NONE', #3778, #429, #3840 ) ;
#2943=VERTEX_POINT ( 'NONE', #676 ) ;
#2945=CARTESIAN_POINT ( 'NONE',  ( -317.5233545270529021, 6.019019530952224355E-15, 141.2297481720574126 ) ) ;
#2955=ORIENTED_EDGE ( 'NONE', *, *, #4038, .T. ) ;
#2957=CARTESIAN_POINT ( 'NONE',  ( -316.5277671734493197, 2.222614453595266735E-15, 141.3235875099962584 ) ) ;
#2958=CYLINDRICAL_SURFACE ( 'NONE', #2829, 4.382543221487789964 ) ;
#2959=CARTESIAN_POINT ( 'NONE',  ( -344.9797493358575480, 2.222614453595284090E-15, 107.5044404032142751 ) ) ;
#2960=CARTESIAN_POINT ( 'NONE',  ( -338.5048350180761076, 2.276824562219559311E-15, 38.80891300457378890 ) ) ;
#2961=AXIS2_PLACEMENT_3D ( 'NONE', #1035, #1889, #1418 ) ;
#2963=CARTESIAN_POINT ( 'NONE',  ( -167.9289969670495282, -24.99999999999981881, 528.5729890193230176 ) ) ;
#2964=CARTESIAN_POINT ( 'NONE',  ( -360.7307227603793649, 2.222614453595284090E-15, 354.4373729494858480 ) ) ;
#2966=ORIENTED_EDGE ( 'NONE', *, *, #1435, .F. ) ;
#2967=ORIENTED_EDGE ( 'NONE', *, *, #1605, .F. ) ;
#2970=AXIS2_PLACEMENT_3D ( 'NONE', #4313, #3575, #541 ) ;
#2972=CYLINDRICAL_SURFACE ( 'NONE', #4085, 4.382543221487789964 ) ;
#2973=VERTEX_POINT ( 'NONE', #701 ) ;
#2978=DIRECTION ( 'NONE',  ( 1.000000000000000000, -5.777789833161702304E-31, 0.000000000000000000 ) ) ;
#2980=ORIENTED_EDGE ( 'NONE', *, *, #2910, .F. ) ;
#2982=EDGE_CURVE ( 'NONE', #249, #2943, #3578, .T. ) ;
#2983=ORIENTED_EDGE ( 'NONE', *, *, #4316, .T. ) ;
#2986=DIRECTION ( 'NONE',  ( 0.09383933793885537722, -2.626968444144180508E-31, -0.9955873536034883786 ) ) ;
#2989=( LENGTH_UNIT ( ) NAMED_UNIT ( * ) SI_UNIT ( .MILLI., .METRE. ) );
#2990=ORIENTED_EDGE ( 'NONE', *, *, #5271, .F. ) ;
#2991=CARTESIAN_POINT ( 'NONE',  ( -339.2542556961718674, -2.870467298361735770E-14, 239.6247169981594141 ) ) ;
#2992=CARTESIAN_POINT ( 'NONE',  ( -213.0979982360503584, 1.517883041479706208E-15, 511.7519955242227070 ) ) ;
#2994=ORIENTED_EDGE ( 'NONE', *, *, #695, .F. ) ;
#3001=CARTESIAN_POINT ( 'NONE',  ( -378.3480224348070351, 2.222614453595300656E-15, 136.5011359113908611 ) ) ;
#3004=CARTESIAN_POINT ( 'NONE',  ( -86.97194166595129161, 3.740497495074990297E-15, 531.0655262460708173 ) ) ;
#3006=CARTESIAN_POINT ( 'NONE',  ( 35.78913469918423829, 0.000000000000000000, 310.6402212931345161 ) ) ;
#3011=ORIENTED_EDGE ( 'NONE', *, *, #4316, .F. ) ;
#3013=VERTEX_POINT ( 'NONE', #1119 ) ;
#3014=LINE ( 'NONE', #2705, #4777 ) ;
#3015=DIRECTION ( 'NONE',  ( 0.9955873536034882676, 0.000000000000000000, 0.09383933793885600172 ) ) ;
#3017=EDGE_CURVE ( 'NONE', #4129, #3237, #3894, .T. ) ;
#3023=CARTESIAN_POINT ( 'NONE',  ( -198.3455225866217404, 1.517883041479706208E-15, 518.3576047634792303 ) ) ;
#3025=CARTESIAN_POINT ( 'NONE',  ( 4.992201166475765284, -24.99999999999981881, 252.6216919286950429 ) ) ;
#3026=CARTESIAN_POINT ( 'NONE',  ( -354.9469840587070735, 2.222614453595298289E-15, 100.5383829474108524 ) ) ;
#3033=( NAMED_UNIT ( * ) PLANE_ANGLE_UNIT ( ) SI_UNIT ( $, .RADIAN. ) );
#3034=AXIS2_PLACEMENT_3D ( 'NONE', #3059, #4269, #1752 ) ;
#3038=CARTESIAN_POINT ( 'NONE',  ( 34.60640066538633874, 2.222614453595284090E-15, 295.6817845355787995 ) ) ;
#3040=CARTESIAN_POINT ( 'NONE',  ( -336.1069982926114221, -24.99999999999981881, 349.6877309229307684 ) ) ;
#3041=CARTESIAN_POINT ( 'NONE',  ( -156.9923520473269321, 0.000000000000000000, 556.8176423728721147 ) ) ;
#3042=DIRECTION ( 'NONE',  ( -0.9955873536034882676, 5.484003909441382024E-31, -0.09383933793885569641 ) ) ;
#3043=AXIS2_PLACEMENT_3D ( 'NONE', #324, #2381, #1998 ) ;
#3045=ORIENTED_EDGE ( 'NONE', *, *, #961, .T. ) ;
#3046=ORIENTED_EDGE ( 'NONE', *, *, #4729, .F. ) ;
#3047=FACE_BOUND ( 'NONE', #1213, .T. ) ;
#3048=CARTESIAN_POINT ( 'NONE',  ( -347.8887688119608015, 2.222614453595284090E-15, 138.3676483649225588 ) ) ;
#3049=LINE ( 'NONE', #4721, #1348 ) ;
#3050=DIRECTION ( 'NONE',  ( -0.09383933793885568253, 2.673190762809473730E-31, 0.9955873536034882676 ) ) ;
#3054=CARTESIAN_POINT ( 'NONE',  ( 31.14585677005056041, -24.99999999999981881, 398.7793066466517757 ) ) ;
#3057=ADVANCED_FACE ( 'NONE', ( #379 ), #2082, .F. ) ;
#3059=CARTESIAN_POINT ( 'NONE',  ( -346.0119820531829191, 0.000000000000000000, 118.4559012928527721 ) ) ;
#3061=ORIENTED_EDGE ( 'NONE', *, *, #3329, .F. ) ;
#3062=CARTESIAN_POINT ( 'NONE',  ( -320.6447527397726276, 2.276824562219559311E-15, 453.8399743637901906 ) ) ;
#3064=CARTESIAN_POINT ( 'NONE',  ( -68.63039925413394826, 1.572093150103981429E-15, 524.1455590405157636 ) ) ;
#3066=CARTESIAN_POINT ( 'NONE',  ( -349.8593949086763928, 2.222614453595284090E-15, 159.2749827905956010 ) ) ;
#3068=VERTEX_POINT ( 'NONE', #814 ) ;
#3073=DIRECTION ( 'NONE',  ( -0.9955873536034883786, 5.496925049605202091E-31, -0.09383933793885522456 ) ) ;
#3077=CARTESIAN_POINT ( 'NONE',  ( -285.5643670724624599, -25.00000000000003197, 494.2304181244473966 ) ) ;
#3078=CARTESIAN_POINT ( 'NONE',  ( -351.6990976162155107, 2.276824562219559311E-15, 238.4517252739237847 ) ) ;
#3081=CARTESIAN_POINT ( 'NONE',  ( -334.2906958041416488, 0.000000000000000000, 430.9840019716568804 ) ) ;
#3085=ORIENTED_EDGE ( 'NONE', *, *, #1605, .T. ) ;
#3086=CARTESIAN_POINT ( 'NONE',  ( 12.58979647763672283, 2.222614453595284090E-15, 97.46177917736021357 ) ) ;
#3088=EDGE_CURVE ( 'NONE', #4329, #911, #5026, .T. ) ;
#3094=UNCERTAINTY_MEASURE_WITH_UNIT (LENGTH_MEASURE( 1.000000000000000082E-05 ), #852, 'distance_accuracy_value', 'NONE');
#3095=VERTEX_POINT ( 'NONE', #1229 ) ;
#3096=CARTESIAN_POINT ( 'NONE',  ( -366.9888585194556754, 2.222614453595296317E-15, 99.40337302301857392 ) ) ;
#3097=CARTESIAN_POINT ( 'NONE',  ( -346.1058213911226176, 0.000000000000000000, 119.4514886464559424 ) ) ;
#3099=DIRECTION ( 'NONE',  ( 0.09383933793885568253, -2.673190762809473730E-31, -0.9955873536034882676 ) ) ;
#3100=VERTEX_POINT ( 'NONE', #4989 ) ;
#3101=AXIS2_PLACEMENT_3D ( 'NONE', #4492, #718, #319 ) ;
#3103=CARTESIAN_POINT ( 'NONE',  ( 11.81831109762766729, -25.00000000000000355, 46.95220429669349471 ) ) ;
#3104=CYLINDRICAL_SURFACE ( 'NONE', #2062, 4.382543221487789964 ) ;
#3105=CIRCLE ( 'NONE', #3794, 27.50000000000126832 ) ;
#3108=AXIS2_PLACEMENT_3D ( 'NONE', #4692, #514, #929 ) ;
#3109=CARTESIAN_POINT ( 'NONE',  ( -347.8887688119603467, 2.222614453595284090E-15, 138.3676483649222178 ) ) ;
#3110=CARTESIAN_POINT ( 'NONE',  ( 24.85474708473287109, 3.252606517456513302E-16, 216.1905617304896623 ) ) ;
#3112=AXIS2_PLACEMENT_3D ( 'NONE', #687, #1510, #3209 ) ;
#3116=CARTESIAN_POINT ( 'NONE',  ( -72.60637664584220374, 25.00000000000018474, 552.9197695054134556 ) ) ;
#3118=ORIENTED_EDGE ( 'NONE', *, *, #1565, .T. ) ;
#3119=AXIS2_PLACEMENT_3D ( 'NONE', #4976, #391, #1216 ) ;
#3120=CIRCLE ( 'NONE', #4954, 28.50000000000127898 ) ;
#3122=AXIS2_PLACEMENT_3D ( 'NONE', #1932, #318, #1164 ) ;
#3123=CARTESIAN_POINT ( 'NONE',  ( -353.4921497144319460, 2.222614453595284090E-15, 38.40071206960160310 ) ) ;
#3124=AXIS2_PLACEMENT_3D ( 'NONE', #3928, #588, #3073 ) ;
#3125=ORIENTED_EDGE ( 'NONE', *, *, #1401, .T. ) ;
#3128=CARTESIAN_POINT ( 'NONE',  ( -349.6717162327985307, 3.252606517456513302E-16, 157.2838080833889194 ) ) ;
#3132=ORIENTED_EDGE ( 'NONE', *, *, #4567, .T. ) ;
#3134=CARTESIAN_POINT ( 'NONE',  ( 35.78913469918393275, -24.99999999999981881, 310.6402212931347435 ) ) ;
#3135=DIRECTION ( 'NONE',  ( -0.09383933793885568253, 2.673190762809473730E-31, 0.9955873536034882676 ) ) ;
#3136=MANIFOLD_SOLID_BREP ( 'Boss-Extrude11', #5419 ) ;
#3137=DIRECTION ( 'NONE',  ( -0.9955873536034882676, 5.502656983963330823E-31, -0.09383933793885547436 ) ) ;
#3138=ADVANCED_FACE ( 'NONE', ( #1827 ), #3812, .T. ) ;
#3139=DIRECTION ( 'NONE',  ( -0.9955873536034883786, 5.430490990731020552E-31, -0.09383933793885548824 ) ) ;
#3140=CARTESIAN_POINT ( 'NONE',  ( -57.28677601057280100, 3.252606517456513302E-16, 546.4981013186296650 ) ) ;
#3142=ORIENTED_EDGE ( 'NONE', *, *, #3827, .T. ) ;
#3143=CARTESIAN_POINT ( 'NONE',  ( -367.0460729392618759, 0.000000000000000000, 268.0688838304710089 ) ) ;
#3147=CLOSED_SHELL ( 'NONE', ( #3057, #3524, #3994, #3175, #3162, #1375 ) ) ;
#3148=ORIENTED_EDGE ( 'NONE', *, *, #560, .T. ) ;
#3149=EDGE_LOOP ( 'NONE', ( #1590, #2544, #361, #1315 ) ) ;
#3151=DIRECTION ( 'NONE',  ( 0.9998833722232041143, -6.779273404243022909E-31, -0.01527226085271993737 ) ) ;
#3155=ADVANCED_FACE ( 'NONE', ( #1309 ), #97, .T. ) ;
#3162=ADVANCED_FACE ( 'NONE', ( #1333 ), #3464, .T. ) ;
#3163=CARTESIAN_POINT ( 'NONE',  ( 31.14585677005082687, 2.222614453595284090E-15, 398.7793066466531968 ) ) ;
#3164=DIRECTION ( 'NONE',  ( 0.09383933793885125552, -2.549931246368697204E-31, -0.9955873536034887117 ) ) ;
#3166=DIRECTION ( 'NONE',  ( -0.9955873536034882676, 5.502656983963330823E-31, -0.09383933793885547436 ) ) ;
#3167=CARTESIAN_POINT ( 'NONE',  ( 11.81831109762766729, 25.00000000000000355, 46.95220429669349471 ) ) ;
#3169=CARTESIAN_POINT ( 'NONE',  ( -35.15684241565268309, -24.99999999999981881, 493.9702760599490716 ) ) ;
#3171=CARTESIAN_POINT ( 'NONE',  ( 8.821273309659243722, 25.00000000000018474, 380.5076279642384520 ) ) ;
#3175=ADVANCED_FACE ( 'NONE', ( #2610, #538 ), #4722, .F. ) ;
#3176=ADVANCED_FACE ( 'NONE', ( #237 ), #264, .T. ) ;
#3177=ORIENTED_EDGE ( 'NONE', *, *, #224, .F. ) ;
#3180=CARTESIAN_POINT ( 'NONE',  ( -338.5986743560152377, 2.276824562219559311E-15, 39.80450035817695209 ) ) ;
#3182=DIRECTION ( 'NONE',  ( 0.9955873536034882676, -5.499791016784056700E-31, 0.09383933793885550212 ) ) ;
#3184=EDGE_LOOP ( 'NONE', ( #1238, #1010 ) ) ;
#3185=EDGE_CURVE ( 'NONE', #229, #1126, #4075, .T. ) ;
#3190=CYLINDRICAL_SURFACE ( 'NONE', #2565, 27.43532828739476415 ) ;
#3196=DIRECTION ( 'NONE',  ( -0.9955873536034882676, 5.452307672560241053E-31, -0.09383933793885547436 ) ) ;
#3197=CARTESIAN_POINT ( 'NONE',  ( -14.89480152442222582, 25.00000000000018474, 508.6517828409982940 ) ) ;
#3199=CARTESIAN_POINT ( 'NONE',  ( -339.2542556961722084, 3.740497495074990297E-15, 239.6247169981598972 ) ) ;
#3200=CARTESIAN_POINT ( 'NONE',  ( -1.533280346156490337, 2.222614453595284090E-15, 488.4857301958385278 ) ) ;
#3203=EDGE_LOOP ( 'NONE', ( #2917, #4911, #1556, #2638 ) ) ;
#3204=CARTESIAN_POINT ( 'NONE',  ( -39.32426838450110296, 25.00000000000018474, 499.4571537926176461 ) ) ;
#3205=VERTEX_POINT ( 'NONE', #1031 ) ;
#3206=CARTESIAN_POINT ( 'NONE',  ( -318.6333298290857101, -1.512095747587092168E-29, 121.0364830861714154 ) ) ;
#3209=DIRECTION ( 'NONE',  ( -0.9998833722232041143, 6.779273404243020281E-31, 0.01527226085271993043 ) ) ;
#3210=ORIENTED_EDGE ( 'NONE', *, *, #756, .T. ) ;
#3211=PRODUCT_DEFINITION ( 'UNKNOWN', '', #1542, #2314 ) ;
#3213=LINE ( 'NONE', #1107, #1074 ) ;
#3214=DIRECTION ( 'NONE',  ( -0.9955873536034882676, 5.498529991225532962E-31, -0.09383933793885550212 ) ) ;
#3215=CARTESIAN_POINT ( 'NONE',  ( -346.1058213911226176, 0.000000000000000000, 119.4514886464559424 ) ) ;
#3216=DIRECTION ( 'NONE',  ( -0.9955873536034883786, 5.498529991225544347E-31, -0.09383933793885444741 ) ) ;
#3219=ORIENTED_EDGE ( 'NONE', *, *, #1689, .T. ) ;
#3220=CARTESIAN_POINT ( 'NONE',  ( -344.1351952944061168, 5.421010862427522170E-17, 98.54415422078321285 ) ) ;
#3224=CYLINDRICAL_SURFACE ( 'NONE', #4023, 4.382543221487789964 ) ;
#3225=CARTESIAN_POINT ( 'NONE',  ( -35.15684241565268309, 25.00000000000018474, 493.9702760599490716 ) ) ;
#3227=CARTESIAN_POINT ( 'NONE',  ( 36.35777514575885760, 2.222614453595284090E-15, 354.7349908125909792 ) ) ;
#3228=DIRECTION ( 'NONE',  ( -0.09383933793885568253, 2.673190762809473730E-31, 0.9955873536034882676 ) ) ;
#3230=CARTESIAN_POINT ( 'NONE',  ( -8.629236981538166873, 25.00000000000000355, 142.6115645898824198 ) ) ;
#3234=DIRECTION ( 'NONE',  ( -0.9998833722232041143, 6.779273404243020281E-31, 0.01527226085271993043 ) ) ;
#3236=VERTEX_POINT ( 'NONE', #2709 ) ;
#3237=VERTEX_POINT ( 'NONE', #4470 ) ;
#3241=CARTESIAN_POINT ( 'NONE',  ( -351.6423423295148041, 5.421010862427522170E-17, 178.1911425090623311 ) ) ;
#3242=AXIS2_PLACEMENT_3D ( 'NONE', #4448, #331, #3196 ) ;
#3243=DIRECTION ( 'NONE',  ( -5.679099018122554920E-31, -1.000000000000000000, 2.149753974990777610E-31 ) ) ;
#3244=ORIENTED_EDGE ( 'NONE', *, *, #275, .F. ) ;
#3246=FACE_OUTER_BOUND ( 'NONE', #842, .T. ) ;
#3248=DIRECTION ( 'NONE',  ( 0.09383933793885536334, -2.626968444144180070E-31, -0.9955873536034882676 ) ) ;
#3249=AXIS2_PLACEMENT_3D ( 'NONE', #2107, #48, #3780 ) ;
#3251=CARTESIAN_POINT ( 'NONE',  ( -323.7051989975983588, 2.222614453595284090E-15, 41.20828864675230108 ) ) ;
#3252=CARTESIAN_POINT ( 'NONE',  ( 0.07030049711781446997, 25.00000000000000355, 219.5055207296751689 ) ) ;
#3253=CARTESIAN_POINT ( 'NONE',  ( -19.78983854945498422, 2.222614453595284090E-15, 515.1268587725810448 ) ) ;
#3255=ORIENTED_EDGE ( 'NONE', *, *, #3355, .T. ) ;
#3256=CARTESIAN_POINT ( 'NONE',  ( -354.3266237013165778, 25.00000000000018474, 381.2801272015587983 ) ) ;
#3258=CARTESIAN_POINT ( 'NONE',  ( -320.2813406910036633, 5.421010862425789758E-17, 181.1470816541363718 ) ) ;
#3259=ADVANCED_FACE ( 'NONE', ( #1053 ), #205, .T. ) ;
#3260=CARTESIAN_POINT ( 'NONE',  ( -374.4264635139651887, 2.571758278209474793E-15, 196.1322634844163417 ) ) ;
#3268=CARTESIAN_POINT ( 'NONE',  ( -319.5145292342597827, 5.712857831165349408E-15, 141.0420694961801189 ) ) ;
#3271=FACE_OUTER_BOUND ( 'NONE', #169, .T. ) ;
#3272=FACE_OUTER_BOUND ( 'NONE', #2254, .T. ) ;
#3278=CARTESIAN_POINT ( 'NONE',  ( -12.39202333278749357, 1.572093150103981429E-15, 98.84296066633379496 ) ) ;
#3279=CARTESIAN_POINT ( 'NONE',  ( -174.3534642324304116, 5.421010862427522170E-17, 552.7876087698471110 ) ) ;
#3280=AXIS2_PLACEMENT_3D ( 'NONE', #3927, #2707, #564 ) ;
#3282=CARTESIAN_POINT ( 'NONE',  ( 0.07030049711781446997, 25.00000000000000355, 219.5055207296751689 ) ) ;
#3284=AXIS2_PLACEMENT_3D ( 'NONE', #779, #3796, #1707 ) ;
#3287=VECTOR ( 'NONE', #2119, 1000.000000000000000 ) ;
#3289=ORIENTED_EDGE ( 'NONE', *, *, #4132, .F. ) ;
#3291=AXIS2_PLACEMENT_3D ( 'NONE', #2032, #5375, #2104 ) ;
#3292=EDGE_LOOP ( 'NONE', ( #1923, #3695, #1524, #436 ) ) ;
#3293=CARTESIAN_POINT ( 'NONE',  ( -351.6990976162155107, 2.276824562219559311E-15, 238.4517252739237847 ) ) ;
#3294=DIRECTION ( 'NONE',  ( -0.9955873536034882676, 5.484003909441392533E-31, -0.09383933793885569641 ) ) ;
#3297=AXIS2_PLACEMENT_3D ( 'NONE', #1547, #4111, #1463 ) ;
#3300=ORIENTED_EDGE ( 'NONE', *, *, #2008, .F. ) ;
#3302=ORIENTED_EDGE ( 'NONE', *, *, #4878, .T. ) ;
#3303=CARTESIAN_POINT ( 'NONE',  ( -353.4252897503525332, 0.000000000000000000, 197.1073022275279243 ) ) ;
#3306=CIRCLE ( 'NONE', #4344, 31.50000000000125766 ) ;
#3311=CARTESIAN_POINT ( 'NONE',  ( 6.585909452840001954, 25.00000000000018474, 393.9228865916072664 ) ) ;
#3312=CARTESIAN_POINT ( 'NONE',  ( -19.78983854945535725, -24.99999999999981881, 515.1268587725797943 ) ) ;
#3314=VERTEX_POINT ( 'NONE', #1081 ) ;
#3315=DIRECTION ( 'NONE',  ( 0.09383933793885537722, -2.626968444144180508E-31, -0.9955873536034883786 ) ) ;
#3321=FACE_OUTER_BOUND ( 'NONE', #497, .T. ) ;
#3322=ORIENTED_EDGE ( 'NONE', *, *, #3827, .F. ) ;
#3323=ORIENTED_EDGE ( 'NONE', *, *, #2852, .F. ) ;
#3329=EDGE_CURVE ( 'NONE', #3835, #251, #1697, .T. ) ;
#3333=EDGE_CURVE ( 'NONE', #251, #3835, #4773, .T. ) ;
#3334=CARTESIAN_POINT ( 'NONE',  ( -80.59222536594906217, 3.740497495074990297E-15, 529.1597157429033587 ) ) ;
#3335=CARTESIAN_POINT ( 'NONE',  ( -299.8611223228771792, 24.99999999999997158, 439.6443911606498887 ) ) ;
#3336=CARTESIAN_POINT ( 'NONE',  ( 5.624351423727524946, 2.222614453595284090E-15, 474.0483466084679662 ) ) ;
#3338=TOROIDAL_SURFACE ( 'NONE', #5335, 28.50000000000115818, 1.000000000000000000 ) ;
#3339=VERTEX_POINT ( 'NONE', #3791 ) ;
#3341=ORIENTED_EDGE ( 'NONE', *, *, #5175, .T. ) ;
#3344=DIRECTION ( 'NONE',  ( 0.09383933793885568253, -2.673190762809473730E-31, -0.9955873536034882676 ) ) ;
#3345=DIRECTION ( 'NONE',  ( 0.9998833722232040033, -6.797399803719615819E-31, -0.01527226085271964420 ) ) ;
#3346=ADVANCED_FACE ( 'NONE', ( #3830 ), #2972, .T. ) ;
#3348=ORIENTED_EDGE ( 'NONE', *, *, #130, .T. ) ;
#3352=DIRECTION ( 'NONE',  ( 0.09383933793885568253, -2.673190762809473730E-31, -0.9955873536034882676 ) ) ;
#3355=EDGE_CURVE ( 'NONE', #2877, #5050, #209, .T. ) ;
#3356=CARTESIAN_POINT ( 'NONE',  ( -35.15684241565247703, 1.843143693225357538E-15, 493.9702760599520275 ) ) ;
#3357=CARTESIAN_POINT ( 'NONE',  ( -0.4023372602957597799, 1.572093150103981429E-15, 421.4664991284013809 ) ) ;
#3359=EDGE_LOOP ( 'NONE', ( #4311, #80, #2717, #190 ) ) ;
#3360=AXIS2_PLACEMENT_3D ( 'NONE', #2683, #2265, #2654 ) ;
#3362=CARTESIAN_POINT ( 'NONE',  ( -318.7271691670245559, -1.485826063145656437E-29, 122.0320704397746709 ) ) ;
#3364=ORIENTED_EDGE ( 'NONE', *, *, #869, .F. ) ;
#3366=AXIS2_PLACEMENT_3D ( 'NONE', #3613, #5270, #3511 ) ;
#3372=AXIS2_PLACEMENT_3D ( 'NONE', #3241, #640, #3182 ) ;
#3374=EDGE_LOOP ( 'NONE', ( #1647, #539, #2076, #2431 ) ) ;
#3379=DIRECTION ( 'NONE',  ( -0.9955873536034882676, 5.452307672560245432E-31, -0.09383933793885568253 ) ) ;
#3385=CARTESIAN_POINT ( 'NONE',  ( 11.35554381053716000, 3.794707603699265519E-15, 353.5846600851142512 ) ) ;
#3386=CARTESIAN_POINT ( 'NONE',  ( -48.20943979674346735, -24.99999999999981881, 509.2978244404901602 ) ) ;
#3391=PLANE ( 'NONE',  #3034 ) ;
#3393=DIRECTION ( 'NONE',  ( 0.09383933793885537722, -2.626968444144180508E-31, -0.9955873536034883786 ) ) ;
#3395=EDGE_LOOP ( 'NONE', ( #2221, #4877 ) ) ;
#3398=EDGE_CURVE ( 'NONE', #8, #2973, #735, .T. ) ;
#3401=DIRECTION ( 'NONE',  ( -0.9955873536034883786, 5.498529991225525955E-31, -0.09383933793885444741 ) ) ;
#3409=DIRECTION ( 'NONE',  ( -0.09383933793885568253, 2.673190762809473730E-31, 0.9955873536034882676 ) ) ;
#3411=DIRECTION ( 'NONE',  ( -0.09383933793885537722, 2.611561004589082621E-31, 0.9955873536034883786 ) ) ;
#3412=ORIENTED_EDGE ( 'NONE', *, *, #1601, .F. ) ;
#3413=CARTESIAN_POINT ( 'NONE',  ( -336.3653681801726520, -1.035187345108139271E-30, 239.8970098219878651 ) ) ;
#3414=CARTESIAN_POINT ( 'NONE',  ( -12.39202333278750601, -25.00000000000000355, 98.84296066633362443 ) ) ;
#3415=CARTESIAN_POINT ( 'NONE',  ( -345.9181427152443007, 2.222614453595284090E-15, 117.4603139392499429 ) ) ;
#3417=EDGE_LOOP ( 'NONE', ( #2268, #2605, #4197, #4174 ) ) ;
#3421=DIRECTION ( 'NONE',  ( -0.9955873536034882676, 5.452307672560245432E-31, -0.09383933793885568253 ) ) ;
#3422=EDGE_LOOP ( 'NONE', ( #4740, #1929, #3255, #1413 ) ) ;
#3425=CARTESIAN_POINT ( 'NONE',  ( -353.5191290882918338, 0.000000000000000000, 198.1028895811323025 ) ) ;
#3426=CARTESIAN_POINT ( 'NONE',  ( 11.65205807320727871, -24.99999999999981881, 340.0738060255407049 ) ) ;
#3427=( NAMED_UNIT ( * ) PLANE_ANGLE_UNIT ( ) SI_UNIT ( $, .RADIAN. ) );
#3428=DIRECTION ( 'NONE',  ( 0.09383933793885537722, -2.626968444144180508E-31, -0.9955873536034883786 ) ) ;
#3429=DIRECTION ( 'NONE',  ( -1.000000000000000000, -1.219242865862094703E-16, 0.000000000000000000 ) ) ;
#3436=CARTESIAN_POINT ( 'NONE',  ( -346.1058213911226176, 0.000000000000000000, 119.4514886464559424 ) ) ;
#3440=CARTESIAN_POINT ( 'NONE',  ( 6.585909452865815084, -24.99999999999981881, 393.9228865916069253 ) ) ;
#3441=DIRECTION ( 'NONE',  ( -0.09383933793885536334, 2.626968444144180070E-31, 0.9955873536034882676 ) ) ;
#3444=ORIENTED_EDGE ( 'NONE', *, *, #2342, .T. ) ;
#3445=CARTESIAN_POINT ( 'NONE',  ( -378.2336344863770705, 2.222614453595299473E-15, 156.6005616593380694 ) ) ;
#3446=ORIENTED_EDGE ( 'NONE', *, *, #4533, .F. ) ;
#3447=CARTESIAN_POINT ( 'NONE',  ( 36.66581985038887126, 25.00000000000018474, 340.1662229844756098 ) ) ;
#3448=ORIENTED_EDGE ( 'NONE', *, *, #4860, .T. ) ;
#3450=CARTESIAN_POINT ( 'NONE',  ( -249.5207023207449879, -25.00000000000003197, 491.2832465756976035 ) ) ;
#3455=ORIENTED_EDGE ( 'NONE', *, *, #3885, .F. ) ;
#3459=CYLINDRICAL_SURFACE ( 'NONE', #741, 4.382543221487789964 ) ;
#3461=DIRECTION ( 'NONE',  ( 0.09383933793885537722, -2.626968444144180508E-31, -0.9955873536034883786 ) ) ;
#3464=CYLINDRICAL_SURFACE ( 'NONE', #3108, 21.00000000000012790 ) ;
#3466=ADVANCED_FACE ( 'NONE', ( #1579 ), #2152, .F. ) ;
#3467=CIRCLE ( 'NONE', #1433, 1.000000000000000888 ) ;
#3468=CARTESIAN_POINT ( 'NONE',  ( -353.3314504124138011, 0.000000000000000000, 196.1117148739250808 ) ) ;
#3469=AXIS2_PLACEMENT_3D ( 'NONE', #1280, #3411, #4258 ) ;
#3470=CARTESIAN_POINT ( 'NONE',  ( -249.5207023207449879, -25.00000000000003197, 491.2832465756976035 ) ) ;
#3471=DIRECTION ( 'NONE',  ( -1.219242865862094703E-16, 1.000000000000000000, -1.149200448409289593E-17 ) ) ;
#3472=AXIS2_PLACEMENT_3D ( 'NONE', #5081, #2260, #2626 ) ;
#3473=VECTOR ( 'NONE', #3441, 1000.000000000000114 ) ;
#3475=ORIENTED_EDGE ( 'NONE', *, *, #1565, .F. ) ;
#3478=AXIS2_PLACEMENT_3D ( 'NONE', #2959, #409, #3379 ) ;
#3481=CARTESIAN_POINT ( 'NONE',  ( -49.96441683051505578, 2.222614453595284090E-15, 542.4422122871075089 ) ) ;
#3482=ORIENTED_EDGE ( 'NONE', *, *, #3333, .T. ) ;
#3485=CARTESIAN_POINT ( 'NONE',  ( -167.9289969670495282, -24.99999999999981881, 528.5729890193230176 ) ) ;
#3489=ORIENTED_EDGE ( 'NONE', *, *, #4050, .T. ) ;
#3490=VERTEX_POINT ( 'NONE', #1701 ) ;
#3492=FACE_OUTER_BOUND ( 'NONE', #1384, .T. ) ;
#3493=CARTESIAN_POINT ( 'NONE',  ( -374.4264635139651887, 2.571758278209474793E-15, 196.1322634844163417 ) ) ;
#3494=ORIENTED_EDGE ( 'NONE', *, *, #1513, .T. ) ;
#3497=CARTESIAN_POINT ( 'NONE',  ( -264.1404626571541598, -25.00000000000003197, 511.7445549721641100 ) ) ;
#3499=EDGE_CURVE ( 'NONE', #5037, #2290, #4343, .T. ) ;
#3500=ADVANCED_FACE ( 'NONE', ( #2409 ), #1833, .T. ) ;
#3502=ORIENTED_EDGE ( 'NONE', *, *, #1401, .F. ) ;
#3503=CARTESIAN_POINT ( 'NONE',  ( -0.8482259245422840710, 2.276824562219559311E-15, 36.14439046289818691 ) ) ;
#3506=AXIS2_PLACEMENT_3D ( 'NONE', #1862, #1478, #3139 ) ;
#3509=CARTESIAN_POINT ( 'NONE',  ( 36.35777514575885760, 2.222614453595284090E-15, 354.7349908125909792 ) ) ;
#3511=DIRECTION ( 'NONE',  ( -0.9998833722232041143, 6.779273404243020281E-31, 0.01527226085271993043 ) ) ;
#3512=CARTESIAN_POINT ( 'NONE',  ( -223.9642223310785312, 5.421010862427522170E-17, 534.3227077389987016 ) ) ;
#3514=TOROIDAL_SURFACE ( 'NONE', #1646, 28.50000000000115818, 1.000000000000000000 ) ;
#3519=DIRECTION ( 'NONE',  ( -0.09383933793885537722, 2.611561004589082621E-31, 0.9955873536034883786 ) ) ;
#3521=DIRECTION ( 'NONE',  ( 0.9998833722232041143, -6.779273404243020281E-31, -0.01527226085271993043 ) ) ;
#3522=CARTESIAN_POINT ( 'NONE',  ( -339.2542556961734590, -24.99999999999981881, 239.6247169981589309 ) ) ;
#3524=ADVANCED_FACE ( 'NONE', ( #4207 ), #2504, .T. ) ;
#3526=CARTESIAN_POINT ( 'NONE',  ( 23.50217280487988347, 25.00000000000018474, 428.9062724124379997 ) ) ;
#3528=EDGE_LOOP ( 'NONE', ( #1484, #3475 ) ) ;
#3529=CARTESIAN_POINT ( 'NONE',  ( -19.78983854945535725, 25.00000000000018474, 515.1268587725797943 ) ) ;
#3532=DIRECTION ( 'NONE',  ( -0.9955873536034882676, 5.406119142139367196E-31, -0.09383933793885596009 ) ) ;
#3534=UNCERTAINTY_MEASURE_WITH_UNIT (LENGTH_MEASURE( 1.000000000000000082E-05 ), #2989, 'distance_accuracy_value', 'NONE');
#3535=EDGE_LOOP ( 'NONE', ( #4455, #3210, #2663, #3446 ) ) ;
#3537=PLANE ( 'NONE',  #1530 ) ;
#3538=CYLINDRICAL_SURFACE ( 'NONE', #807, 4.382543221487789964 ) ;
#3541=VERTEX_POINT ( 'NONE', #2940 ) ;
#3543=CARTESIAN_POINT ( 'NONE',  ( -122.4270646331732451, -24.99999999999981881, 560.5113017241552598 ) ) ;
#3544=FACE_OUTER_BOUND ( 'NONE', #3203, .T. ) ;
#3546=AXIS2_PLACEMENT_3D ( 'NONE', #5363, #1599, #397 ) ;
#3550=CARTESIAN_POINT ( 'NONE',  ( -0.6802310551622114954, 2.222614453595284090E-15, 47.14310755735262859 ) ) ;
#3551=CARTESIAN_POINT ( 'NONE',  ( 31.14585677005056041, 25.00000000000018474, 398.7793066466517757 ) ) ;
#3555=CARTESIAN_POINT ( 'NONE',  ( -105.2090356704102447, 25.00000000000018474, 560.1816718768288865 ) ) ;
#3558=LINE ( 'NONE', #3206, #464 ) ;
#3559=CIRCLE ( 'NONE', #3122, 27.43532828739476415 ) ;
#3566=ADVANCED_FACE ( 'NONE', ( #1662 ), #2315, .T. ) ;
#3573=EDGE_LOOP ( 'NONE', ( #5384, #1971 ) ) ;
#3575=DIRECTION ( 'NONE',  ( 0.09383933793885568253, -2.673190762809473730E-31, -0.9955873536034882676 ) ) ;
#3576=CARTESIAN_POINT ( 'NONE',  ( 33.59898979596731294, 5.421010862427522170E-17, 384.0431050523496310 ) ) ;
#3578=LINE ( 'NONE', #1560, #1514 ) ;
#3579=CARTESIAN_POINT ( 'NONE',  ( -347.9826081498995336, 2.222614453595284090E-15, 139.3632357185260560 ) ) ;
#3581=CARTESIAN_POINT ( 'NONE',  ( 34.60640066538617532, 25.00000000000018474, 295.6817845355782879 ) ) ;
#3583=CARTESIAN_POINT ( 'NONE',  ( 29.77542608467487995, -25.00000000000000355, 249.2409987768023711 ) ) ;
#3585=CARTESIAN_POINT ( 'NONE',  ( 8.821273309647297722, 3.740497495074990297E-15, 380.5076279642372015 ) ) ;
#3588=CARTESIAN_POINT ( 'NONE',  ( -317.7315818134219398, 3.490243377570107522E-15, 122.1259097777134457 ) ) ;
#3589=EDGE_LOOP ( 'NONE', ( #1886, #5016 ) ) ;
#3591=ORIENTED_EDGE ( 'NONE', *, *, #798, .T. ) ;
#3594=AXIS2_PLACEMENT_3D ( 'NONE', #1148, #2862, #2004 ) ;
#3599=VERTEX_POINT ( 'NONE', #901 ) ;
#3603=CARTESIAN_POINT ( 'NONE',  ( -349.7655555707375470, 2.222614453595284090E-15, 158.2793954369922176 ) ) ;
#3604=CARTESIAN_POINT ( 'NONE',  ( -347.9826081498995336, 2.222614453595284090E-15, 139.3632357185260560 ) ) ;
#3605=CARTESIAN_POINT ( 'NONE',  ( -348.7799179161582970, -14.95948628165117178, 101.1196613272007738 ) ) ;
#3606=CARTESIAN_POINT ( 'NONE',  ( 36.35777514575885760, 2.222614453595284090E-15, 354.7349908125909792 ) ) ;
#3608=CARTESIAN_POINT ( 'NONE',  ( -13.17877320795229856, -25.00000000000000355, 47.33401081801169141 ) ) ;
#3609=CARTESIAN_POINT ( 'NONE',  ( -30.63277980166695258, 0.000000000000000000, 527.1358351633697339 ) ) ;
#3611=CARTESIAN_POINT ( 'NONE',  ( -80.59222536594943165, 25.00000000000018474, 529.1597157429057461 ) ) ;
#3612=EDGE_LOOP ( 'NONE', ( #875, #2262 ) ) ;
#3613=CARTESIAN_POINT ( 'NONE',  ( -0.8482259245422840710, 2.276824562219559311E-15, 36.14439046289818691 ) ) ;
#3615=EDGE_CURVE ( 'NONE', #4307, #4331, #3990, .T. ) ;
#3619=DIRECTION ( 'NONE',  ( 0.09383933793885568253, -2.673190762809473730E-31, -0.9955873536034882676 ) ) ;
#3620=DIRECTION ( 'NONE',  ( -0.9955873536034882676, 5.452307672560243681E-31, -0.09383933793885551600 ) ) ;
#3623=AXIS2_PLACEMENT_3D ( 'NONE', #3048, #4360, #587 ) ;
#3625=PLANE ( 'NONE',  #4341 ) ;
#3626=CARTESIAN_POINT ( 'NONE',  ( -207.8397519515728504, 5.421010862427522170E-17, 541.5412455041541762 ) ) ;
#3627=CYLINDRICAL_SURFACE ( 'NONE', #2506, 31.50000000000114397 ) ;
#3629=EDGE_CURVE ( 'NONE', #278, #3745, #1749, .T. ) ;
#3634=CARTESIAN_POINT ( 'NONE',  ( -121.8424039467700055, 25.00000000000018474, 535.4314447305361000 ) ) ;
#3636=CARTESIAN_POINT ( 'NONE',  ( 34.60640066538633874, 2.222614453595284090E-15, 295.6817845355787995 ) ) ;
#3637=CARTESIAN_POINT ( 'NONE',  ( -367.0882437885061904, 2.222614453595284090E-15, 297.8351940652699454 ) ) ;
#3640=CARTESIAN_POINT ( 'NONE',  ( -285.5643670724624599, 24.99999999999997158, 494.2304181244473966 ) ) ;
#3643=MECHANICAL_DESIGN_GEOMETRIC_PRESENTATION_REPRESENTATION('',(#1521),#4513);
#3650=VERTEX_POINT ( 'NONE', #3026 ) ;
#3659=CARTESIAN_POINT ( 'NONE',  ( -367.0882437885061904, 2.222614453595284090E-15, 297.8351940652699454 ) ) ;
#3662=EDGE_CURVE ( 'NONE', #1126, #229, #1791, .T. ) ;
#3663=CARTESIAN_POINT ( 'NONE',  ( -357.8553543223658835, 2.759321206427282701E-15, 37.98945711520877211 ) ) ;
#3664=CARTESIAN_POINT ( 'NONE',  ( -207.8397519515722252, 24.99999999999997158, 541.5412455041529256 ) ) ;
#3665=CARTESIAN_POINT ( 'NONE',  ( 33.59898979596731294, 5.421010862427522170E-17, 384.0431050523496310 ) ) ;
#3669=CARTESIAN_POINT ( 'NONE',  ( -360.7307227603797060, 25.00000000000018474, 354.4373729494859049 ) ) ;
#3672=CARTESIAN_POINT ( 'NONE',  ( -319.3419943896644213, 2.222614453595281723E-15, 41.61954360114513207 ) ) ;
#3674=VERTEX_POINT ( 'NONE', #2637 ) ;
#3676=DIRECTION ( 'NONE',  ( -0.9955873536034882676, 5.502656983963329947E-31, -0.09383933793885568253 ) ) ;
#3677=DIRECTION ( 'NONE',  ( -1.000000000000000000, -1.219242865862092731E-16, 0.000000000000000000 ) ) ;
#3680=VERTEX_POINT ( 'NONE', #3953 ) ;
#3683=CARTESIAN_POINT ( 'NONE',  ( 16.31778627263218695, 2.276824562219550240E-15, 46.88347912285639296 ) ) ;
#3686=CARTESIAN_POINT ( 'NONE',  ( -334.2906958041451162, 24.99999999999997158, 430.9840019716597226 ) ) ;
#3689=CARTESIAN_POINT ( 'NONE',  ( -367.0882437885064746, -24.99999999999981881, 297.8351940652706276 ) ) ;
#3690=ORIENTED_EDGE ( 'NONE', *, *, #78, .T. ) ;
#3691=CARTESIAN_POINT ( 'NONE',  ( -223.9642223310802649, 24.99999999999997158, 534.3227077390027944 ) ) ;
#3693=DIRECTION ( 'NONE',  ( -0.09383933793885536334, 2.611561004589082183E-31, 0.9955873536034882676 ) ) ;
#3695=ORIENTED_EDGE ( 'NONE', *, *, #4226, .T. ) ;
#3698=DIRECTION ( 'NONE',  ( -0.9955873536034883786, 5.452307672560241053E-31, -0.09383933793885559926 ) ) ;
#3702=VERTEX_POINT ( 'NONE', #4749 ) ;
#3704=DIRECTION ( 'NONE',  ( 0.09383933793885568253, -2.673190762809473730E-31, -0.9955873536034882676 ) ) ;
#3705=CARTESIAN_POINT ( 'NONE',  ( -105.2090356704105147, 2.222614453595284090E-15, 560.1816718768288865 ) ) ;
#3706=LINE ( 'NONE', #5373, #2413 ) ;
#3709=CARTESIAN_POINT ( 'NONE',  ( -336.1069982926114221, 25.00000000000018474, 349.6877309229307684 ) ) ;
#3710=CARTESIAN_POINT ( 'NONE',  ( 16.26935751051944479, 3.252606517456513302E-16, 140.3055424402290896 ) ) ;
#3711=AXIS2_PLACEMENT_3D ( 'NONE', #5423, #4201, #43 ) ;
#3712=ORIENTED_EDGE ( 'NONE', *, *, #1206, .F. ) ;
#3713=EDGE_LOOP ( 'NONE', ( #2025, #1406 ) ) ;
#3715=CYLINDRICAL_SURFACE ( 'NONE', #830, 12.50000000000003197 ) ;
#3716=AXIS2_PLACEMENT_3D ( 'NONE', #3425, #30, #1354 ) ;
#3727=ADVANCED_FACE ( 'NONE', ( #1400 ), #2294, .T. ) ;
#3728=AXIS2_PLACEMENT_3D ( 'NONE', #3066, #4275, #3042 ) ;
#3732=EDGE_LOOP ( 'NONE', ( #4164, #2392 ) ) ;
#3733=EDGE_CURVE ( 'NONE', #2554, #3745, #5039, .T. ) ;
#3736=VECTOR ( 'NONE', #1714, 1000.000000000000114 ) ;
#3737=CARTESIAN_POINT ( 'NONE',  ( -375.1735816981183689, 3.367778697655406295E-15, 134.7914792180005179 ) ) ;
#3739=CIRCLE ( 'NONE', #1360, 27.50000000000126832 ) ;
#3743=CARTESIAN_POINT ( 'NONE',  ( 4.992201166475890517, 1.572093150103981429E-15, 252.6216919286947586 ) ) ;
#3744=CARTESIAN_POINT ( 'NONE',  ( 18.31346110193259946, -24.99999999999981881, 444.2932575970297648 ) ) ;
#3745=VERTEX_POINT ( 'NONE', #158 ) ;
#3747=CARTESIAN_POINT ( 'NONE',  ( -353.4252897503525332, 0.000000000000000000, 197.1073022275279243 ) ) ;
#3754=ADVANCED_FACE ( 'NONE', ( #3544 ), #3104, .T. ) ;
#3755=DIRECTION ( 'NONE',  ( 0.9955873536034882676, -5.498529991225536465E-31, 0.09383933793885551600 ) ) ;
#3757=ORIENTED_EDGE ( 'NONE', *, *, #2583, .T. ) ;
#3758=DIRECTION ( 'NONE',  ( -0.09383933793885536334, 2.626968444144180070E-31, 0.9955873536034882676 ) ) ;
#3762=AXIS2_PLACEMENT_3D ( 'NONE', #1893, #4731, #4317 ) ;
#3763=CARTESIAN_POINT ( 'NONE',  ( -249.5207023207451300, 1.843143693225357538E-15, 491.2832465756980014 ) ) ;
#3764=CARTESIAN_POINT ( 'NONE',  ( -121.8424039466566313, 3.794707603699265519E-15, 535.4314447305365547 ) ) ;
#3767=CYLINDRICAL_SURFACE ( 'NONE', #1317, 17.00000000000009948 ) ;
#3769=VERTEX_POINT ( 'NONE', #4775 ) ;
#3778=CARTESIAN_POINT ( 'NONE',  ( -344.4167133082243595, 2.222614453595284090E-15, 101.5309162815936048 ) ) ;
#3780=DIRECTION ( 'NONE',  ( -0.9955873536034882676, 5.456801509096969733E-31, -0.09383933793885547436 ) ) ;
#3781=CARTESIAN_POINT ( 'NONE',  ( -35.15684241565247703, 1.843143693225357538E-15, 493.9702760599520275 ) ) ;
#3784=EDGE_CURVE ( 'NONE', #2195, #3205, #5127, .T. ) ;
#3787=CARTESIAN_POINT ( 'NONE',  ( -319.4001412858301592, 4.060433389145185367E-15, 161.1414952441278956 ) ) ;
#3788=PLANE ( 'NONE',  #2143 ) ;
#3790=ORIENTED_EDGE ( 'NONE', *, *, #85, .F. ) ;
#3791=CARTESIAN_POINT ( 'NONE',  ( -325.1600333418735431, 2.222614453595298289E-15, 103.3459595245619198 ) ) ;
#3793=CARTESIAN_POINT ( 'NONE',  ( -347.7949294740212736, 2.222614453595284090E-15, 137.3720610113191469 ) ) ;
#3794=AXIS2_PLACEMENT_3D ( 'NONE', #1454, #4067, #5262 ) ;
#3795=DIRECTION ( 'NONE',  ( 0.09383933793885568253, -2.673190762809473730E-31, -0.9955873536034882676 ) ) ;
#3796=DIRECTION ( 'NONE',  ( 0.09383933793885537722, -2.626968444144180508E-31, -0.9955873536034883786 ) ) ;
#3797=CYLINDRICAL_SURFACE ( 'NONE', #4950, 12.50000000000009237 ) ;
#3798=VECTOR ( 'NONE', #3693, 1000.000000000000114 ) ;
#3800=AXIS2_PLACEMENT_3D ( 'NONE', #2564, #2159, #480 ) ;
#3806=DIRECTION ( 'NONE',  ( -1.219242865862094703E-16, 1.000000000000000000, -1.149200448409289593E-17 ) ) ;
#3808=ADVANCED_FACE ( 'NONE', ( #760 ), #4260, .F. ) ;
#3809=LINE ( 'NONE', #44, #3736 ) ;
#3810=AXIS2_PLACEMENT_3D ( 'NONE', #401, #2923, #839 ) ;
#3811=AXIS2_PLACEMENT_3D ( 'NONE', #1167, #1729, #4900 ) ;
#3812=CYLINDRICAL_SURFACE ( 'NONE', #3469, 31.50000000000125766 ) ;
#3817=CARTESIAN_POINT ( 'NONE',  ( -342.0244061588616091, 3.740497495074990297E-15, 297.0039604601894894 ) ) ;
#3818=CARTESIAN_POINT ( 'NONE',  ( 10.82492224058167984, 3.740497495074990297E-15, 312.2165827548582229 ) ) ;
#3821=EDGE_CURVE ( 'NONE', #3095, #1738, #4124, .T. ) ;
#3822=ORIENTED_EDGE ( 'NONE', *, *, #365, .F. ) ;
#3824=ORIENTED_EDGE ( 'NONE', *, *, #1034, .F. ) ;
#3825=FACE_OUTER_BOUND ( 'NONE', #4240, .T. ) ;
#3827=EDGE_CURVE ( 'NONE', #3100, #3205, #3706, .T. ) ;
#3830=FACE_OUTER_BOUND ( 'NONE', #4276, .T. ) ;
#3832=CARTESIAN_POINT ( 'NONE',  ( -342.0244061588616091, -24.99999999999981881, 297.0039604601892620 ) ) ;
#3834=CARTESIAN_POINT ( 'NONE',  ( -317.6171938649919753, 5.957787190994850470E-15, 142.2253355256612508 ) ) ;
#3835=VERTEX_POINT ( 'NONE', #700 ) ;
#3837=ORIENTED_EDGE ( 'NONE', *, *, #3333, .F. ) ;
#3838=LINE ( 'NONE', #2957, #2858 ) ;
#3840=DIRECTION ( 'NONE',  ( -0.9955873536034882676, 5.436595176548168253E-31, -0.09383933793885573804 ) ) ;
#3842=VERTEX_POINT ( 'NONE', #1146 ) ;
#3843=CARTESIAN_POINT ( 'NONE',  ( -213.0979982360503584, 1.517883041479706208E-15, 511.7519955242227070 ) ) ;
#3844=CARTESIAN_POINT ( 'NONE',  ( -68.63039925413373510, -24.99999999999981881, 524.1455590405155363 ) ) ;
#3845=DIRECTION ( 'NONE',  ( -0.9955873536034882676, 5.502656983963321189E-31, -0.09383933793885568253 ) ) ;
#3846=EDGE_LOOP ( 'NONE', ( #1716, #3341, #1082, #4495 ) ) ;
#3847=ADVANCED_FACE ( 'NONE', ( #4150, #2857 ), #2769, .T. ) ;
#3849=DIRECTION ( 'NONE',  ( 0.01527226085271972227, 2.095411779493299033E-31, 0.9998833722232041143 ) ) ;
#3852=CARTESIAN_POINT ( 'NONE',  ( -14.89480152442229688, 0.000000000000000000, 508.6517828409968729 ) ) ;
#3855=CARTESIAN_POINT ( 'NONE',  ( -39.32426838447570816, -24.99999999999981881, 499.4571537926179872 ) ) ;
#3856=CARTESIAN_POINT ( 'NONE',  ( -57.28677601057280100, 3.252606517456513302E-16, 546.4981013186296650 ) ) ;
#3857=CARTESIAN_POINT ( 'NONE',  ( -380.0165819072154818, 2.222614453595300261E-15, 175.5167213778050552 ) ) ;
#3859=EDGE_LOOP ( 'NONE', ( #1153, #3444 ) ) ;
#3860=EDGE_LOOP ( 'NONE', ( #5274, #2865 ) ) ;
#3863=DIRECTION ( 'NONE',  ( -0.09383933793885568253, 2.673190762809473730E-31, 0.9955873536034882676 ) ) ;
#3867=VECTOR ( 'NONE', #851, 1000.000000000000114 ) ;
#3870=CARTESIAN_POINT ( 'NONE',  ( -268.5984117390374877, 3.740497495074990297E-15, 475.6392848759629715 ) ) ;
#3872=ORIENTED_EDGE ( 'NONE', *, *, #1692, .F. ) ;
#3873=ORIENTED_EDGE ( 'NONE', *, *, #1030, .F. ) ;
#3875=VERTEX_POINT ( 'NONE', #2824 ) ;
#3876=CARTESIAN_POINT ( 'NONE',  ( -122.4270646331731598, 3.252606517456513302E-16, 560.5113017241549187 ) ) ;
#3879=CARTESIAN_POINT ( 'NONE',  ( 6.585909452865815084, -24.99999999999981881, 393.9228865916069253 ) ) ;
#3880=CARTESIAN_POINT ( 'NONE',  ( 5.624351423727524946, 2.222614453595284090E-15, 474.0483466084679662 ) ) ;
#3885=EDGE_CURVE ( 'NONE', #2041, #4435, #3120, .T. ) ;
#3888=ORIENTED_EDGE ( 'NONE', *, *, #1207, .F. ) ;
#3889=FACE_OUTER_BOUND ( 'NONE', #1709, .T. ) ;
#3890=EDGE_CURVE ( 'NONE', #3314, #3599, #4695, .T. ) ;
#3893=EDGE_CURVE ( 'NONE', #5050, #4617, #481, .T. ) ;
#3894=CIRCLE ( 'NONE', #2925, 4.382543221487789964 ) ;
#3896=DIRECTION ( 'NONE',  ( -0.9955873536034882676, 5.498529991225538217E-31, -0.09383933793885536334 ) ) ;
#3898=AXIS2_PLACEMENT_3D ( 'NONE', #4545, #1263, #2039 ) ;
#3899=DIRECTION ( 'NONE',  ( 0.09383933793885568253, -2.673190762809473730E-31, -0.9955873536034882676 ) ) ;
#3901=CARTESIAN_POINT ( 'NONE',  ( 5.624351423727524946, 2.222614453595284090E-15, 474.0483466084679662 ) ) ;
#3906=CARTESIAN_POINT ( 'NONE',  ( -30.63277980166695258, 0.000000000000000000, 527.1358351633697339 ) ) ;
#3909=CIRCLE ( 'NONE', #1364, 1.000000000000000888 ) ;
#3912=ADVANCED_FACE ( 'NONE', ( #1495 ), #3627, .T. ) ;
#3913=ORIENTED_EDGE ( 'NONE', *, *, #4993, .T. ) ;
#3914=CARTESIAN_POINT ( 'NONE',  ( -156.9923520473269321, 0.000000000000000000, 556.8176423728721147 ) ) ;
#3915=VERTEX_POINT ( 'NONE', #1976 ) ;
#3921=ORIENTED_EDGE ( 'NONE', *, *, #3890, .F. ) ;
#3922=ORIENTED_EDGE ( 'NONE', *, *, #2274, .T. ) ;
#3926=FACE_OUTER_BOUND ( 'NONE', #2728, .T. ) ;
#3927=CARTESIAN_POINT ( 'NONE',  ( -376.2835570001519159, 2.222614453595300656E-15, 114.5982141321147196 ) ) ;
#3928=CARTESIAN_POINT ( 'NONE',  ( -357.2727026058461206, 5.421010862427522170E-17, 237.9263837252718758 ) ) ;
#3929=AXIS2_PLACEMENT_3D ( 'NONE', #824, #5357, #2067 ) ;
#3930=EDGE_LOOP ( 'NONE', ( #2441, #2784, #4956, #2678 ) ) ;
#3932=CARTESIAN_POINT ( 'NONE',  ( -30.63277980166709114, -24.99999999999981881, 527.1358351633700750 ) ) ;
#3935=CARTESIAN_POINT ( 'NONE',  ( 36.66581985038869362, 3.252606517456513302E-16, 340.1662229844753256 ) ) ;
#3937=ORIENTED_EDGE ( 'NONE', *, *, #130, .F. ) ;
#3938=CARTESIAN_POINT ( 'NONE',  ( -14.89480152442222582, 25.00000000000018474, 508.6517828409982940 ) ) ;
#3939=ORIENTED_EDGE ( 'NONE', *, *, #1635, .T. ) ;
#3941=DIRECTION ( 'NONE',  ( -0.9955873536034881566, 5.462637660443544243E-31, -0.09383933793885600172 ) ) ;
#3942=CARTESIAN_POINT ( 'NONE',  ( -347.8887688119608015, 2.222614453595284090E-15, 138.3676483649225588 ) ) ;
#3944=EDGE_LOOP ( 'NONE', ( #3913, #5356 ) ) ;
#3945=ORIENTED_EDGE ( 'NONE', *, *, #983, .F. ) ;
#3947=FACE_OUTER_BOUND ( 'NONE', #3417, .T. ) ;
#3948=CARTESIAN_POINT ( 'NONE',  ( -366.9888585194556754, 2.222614453595296317E-15, 99.40337302301858813 ) ) ;
#3952=CARTESIAN_POINT ( 'NONE',  ( 34.60640066538617532, -24.99999999999981881, 295.6817845355782879 ) ) ;
#3953=CARTESIAN_POINT ( 'NONE',  ( -339.2542556961718674, -2.870467298361735770E-14, 239.6247169981594141 ) ) ;
#3955=AXIS2_PLACEMENT_3D ( 'NONE', #1706, #3344, #5002 ) ;
#3957=CARTESIAN_POINT ( 'NONE',  ( -322.3869033466408496, 2.222614453595269101E-15, 160.8599772303116140 ) ) ;
#3958=CARTESIAN_POINT ( 'NONE',  ( 18.31346110193232590, 2.222614453595284090E-15, 444.2932575970293101 ) ) ;
#3961=EDGE_LOOP ( 'NONE', ( #3757, #1158 ) ) ;
#3962=CARTESIAN_POINT ( 'NONE',  ( 16.26935751051944479, 3.252606517456513302E-16, 140.3055424402290896 ) ) ;
#3963=ORIENTED_EDGE ( 'NONE', *, *, #2515, .F. ) ;
#3966=ORIENTED_EDGE ( 'NONE', *, *, #2518, .T. ) ;
#3967=ORIENTED_EDGE ( 'NONE', *, *, #156, .T. ) ;
#3968=PLANE ( 'NONE',  #2323 ) ;
#3973=CIRCLE ( 'NONE', #3101, 30.50000000000113332 ) ;
#3976=FACE_OUTER_BOUND ( 'NONE', #5383, .T. ) ;
#3977=CARTESIAN_POINT ( 'NONE',  ( 35.78913469918423829, 0.000000000000000000, 310.6402212931345161 ) ) ;
#3984=VERTEX_POINT ( 'NONE', #5041 ) ;
#3985=CARTESIAN_POINT ( 'NONE',  ( -264.1404626571534777, 2.222614453595284090E-15, 511.7445549721628595 ) ) ;
#3987=CARTESIAN_POINT ( 'NONE',  ( 16.26935751051938439, -25.00000000000000355, 140.3055424402287770 ) ) ;
#3988=( GEOMETRIC_REPRESENTATION_CONTEXT ( 3 ) GLOBAL_UNCERTAINTY_ASSIGNED_CONTEXT ( ( #2372 ) ) GLOBAL_UNIT_ASSIGNED_CONTEXT ( ( #4402, #2311, #2836 ) ) REPRESENTATION_CONTEXT ( 'NONE', 'WORKASPACE' ) );
#3990=CIRCLE ( 'NONE', #2755, 27.43532828739476415 ) ;
#3992=CARTESIAN_POINT ( 'NONE',  ( 9.699276322990401766, 25.00000000000018474, 297.8714164406044915 ) ) ;
#3994=ADVANCED_FACE ( 'NONE', ( #4610, #1681 ), #5091, .T. ) ;
#3995=AXIS2_PLACEMENT_3D ( 'NONE', #1089, #1529, #1944 ) ;
#3996=DIRECTION ( 'NONE',  ( -1.000000000000000000, -1.219242865862094703E-16, 0.000000000000000000 ) ) ;
#3997=AXIS2_PLACEMENT_3D ( 'NONE', #4719, #2681, #2286 ) ;
#3998=MECHANICAL_DESIGN_GEOMETRIC_PRESENTATION_REPRESENTATION('',(#4778),#5131);
#4000=EDGE_LOOP ( 'NONE', ( #3837, #2466, #3148, #1842 ) ) ;
#4006=CARTESIAN_POINT ( 'NONE',  ( -351.7361816674535362, 5.421010862427522170E-17, 179.1867298626658283 ) ) ;
#4010=CARTESIAN_POINT ( 'NONE',  ( -347.9826081498995336, 2.222614453595284090E-15, 139.3632357185260560 ) ) ;
#4011=CARTESIAN_POINT ( 'NONE',  ( -19.78983854945498422, 2.222614453595284090E-15, 515.1268587725810448 ) ) ;
#4015=CARTESIAN_POINT ( 'NONE',  ( 16.26935751051944479, 3.252606517456513302E-16, 140.3055424402290896 ) ) ;
#4017=CARTESIAN_POINT ( 'NONE',  ( -198.3455225866217404, 1.517883041479706208E-15, 518.3576047634792303 ) ) ;
#4019=CARTESIAN_POINT ( 'NONE',  ( -198.3455225866221667, 24.99999999999997158, 518.3576047634796851 ) ) ;
#4020=ORIENTED_EDGE ( 'NONE', *, *, #129, .T. ) ;
#4023=AXIS2_PLACEMENT_3D ( 'NONE', #2798, #1563, #677 ) ;
#4028=CARTESIAN_POINT ( 'NONE',  ( -353.3314504124138011, 0.000000000000000000, 196.1117148739250808 ) ) ;
#4029=ADVANCED_FACE ( 'NONE', ( #4254 ), #1446, .F. ) ;
#4031=FACE_OUTER_BOUND ( 'NONE', #5134, .T. ) ;
#4033=CARTESIAN_POINT ( 'NONE',  ( -349.7655555707380017, 2.222614453595284090E-15, 158.2793954369929850 ) ) ;
#4038=EDGE_CURVE ( 'NONE', #936, #3100, #394, .T. ) ;
#4040=CARTESIAN_POINT ( 'NONE',  ( -285.5643670724624599, 24.99999999999997158, 494.2304181244473966 ) ) ;
#4042=CARTESIAN_POINT ( 'NONE',  ( -30.63277980166709114, -24.99999999999981881, 527.1358351633700750 ) ) ;
#4043=CARTESIAN_POINT ( 'NONE',  ( 31.14585677005082687, 2.222614453595284090E-15, 398.7793066466531968 ) ) ;
#4045=CARTESIAN_POINT ( 'NONE',  ( -299.8611223228771792, 24.99999999999997158, 439.6443911606498887 ) ) ;
#4046=AXIS2_PLACEMENT_3D ( 'NONE', #4652, #4958, #2514 ) ;
#4047=ORIENTED_EDGE ( 'NONE', *, *, #2102, .T. ) ;
#4049=DIRECTION ( 'NONE',  ( -0.09383933793885536334, 2.611561004589082183E-31, 0.9955873536034882676 ) ) ;
#4050=EDGE_CURVE ( 'NONE', #3984, #1903, #376, .T. ) ;
#4051=ORIENTED_EDGE ( 'NONE', *, *, #1207, .T. ) ;
#4053=CYLINDRICAL_SURFACE ( 'NONE', #5032, 21.00000000000124700 ) ;
#4055=CARTESIAN_POINT ( 'NONE',  ( -334.2354697480813002, 14.95948628165116823, 40.21575531256979019 ) ) ;
#4057=EDGE_CURVE ( 'NONE', #1390, #3339, #2903, .T. ) ;
#4058=EDGE_LOOP ( 'NONE', ( #2511, #1133 ) ) ;
#4061=ADVANCED_FACE ( 'NONE', ( #1279 ), #4582, .F. ) ;
#4063=DIRECTION ( 'NONE',  ( -0.9955873536034882676, 5.498835694391114214E-31, -0.09383933793885536334 ) ) ;
#4065=CARTESIAN_POINT ( 'NONE',  ( -320.6447527397726276, 2.276824562219559311E-15, 453.8399743637901906 ) ) ;
#4066=DIRECTION ( 'NONE',  ( -0.01527226085271972227, -2.080004339938201584E-31, -0.9998833722232041143 ) ) ;
#4067=DIRECTION ( 'NONE',  ( -0.09383933793885568253, 2.673190762809473730E-31, 0.9955873536034882676 ) ) ;
#4068=AXIS2_PLACEMENT_3D ( 'NONE', #2209, #477, #2155 ) ;
#4069=DIRECTION ( 'NONE',  ( 0.9955873536034882676, -5.273458392682099492E-31, 0.09383933793885600172 ) ) ;
#4071=CARTESIAN_POINT ( 'NONE',  ( -8.629236981538166873, 25.00000000000000355, 142.6115645898824198 ) ) ;
#4072=CARTESIAN_POINT ( 'NONE',  ( -334.2906958041451162, -25.00000000000003197, 430.9840019716597226 ) ) ;
#4073=LINE ( 'NONE', #705, #2744 ) ;
#4075=CIRCLE ( 'NONE', #4944, 4.382543221487789076 ) ;
#4077=CARTESIAN_POINT ( 'NONE',  ( 4.992201166475890517, 1.572093150103981429E-15, 252.6216919286947586 ) ) ;
#4078=VERTEX_POINT ( 'NONE', #1658 ) ;
#4079=DIRECTION ( 'NONE',  ( 0.9955873536034883786, -5.498529991225525955E-31, 0.09383933793885444741 ) ) ;
#4081=( GEOMETRIC_REPRESENTATION_CONTEXT ( 3 ) GLOBAL_UNCERTAINTY_ASSIGNED_CONTEXT ( ( #3534 ) ) GLOBAL_UNIT_ASSIGNED_CONTEXT ( ( #2989, #151, #4662 ) ) REPRESENTATION_CONTEXT ( 'NONE', 'WORKASPACE' ) );
#4085=AXIS2_PLACEMENT_3D ( 'NONE', #2559, #4649, #781 ) ;
#4086=CIRCLE ( 'NONE', #4604, 28.50000000000127542 ) ;
#4089=DIRECTION ( 'NONE',  ( 0.09383933793885568253, -2.673190762809473730E-31, -0.9955873536034882676 ) ) ;
#4092=VECTOR ( 'NONE', #5424, 1000.000000000000114 ) ;
#4094=DIRECTION ( 'NONE',  ( -0.9955873536034882676, 5.273458392682099492E-31, -0.09383933793885600172 ) ) ;
#4096=EDGE_CURVE ( 'NONE', #3490, #2943, #1532, .T. ) ;
#4099=CARTESIAN_POINT ( 'NONE',  ( -347.8887688119603467, 2.222614453595284090E-15, 138.3676483649222178 ) ) ;
#4100=DIRECTION ( 'NONE',  ( -0.9955873536034882676, 5.406119142139367196E-31, -0.09383933793885596009 ) ) ;
#4104=CARTESIAN_POINT ( 'NONE',  ( -5.157059352427092236, 25.00000000000018474, 435.5986320196304860 ) ) ;
#4105=CARTESIAN_POINT ( 'NONE',  ( -122.4270646331731598, 3.252606517456513302E-16, 560.5113017241549187 ) ) ;
#4107=CARTESIAN_POINT ( 'NONE',  ( -320.6447527397745034, 24.99999999999997158, 453.8399743637903612 ) ) ;
#4108=AXIS2_PLACEMENT_3D ( 'NONE', #5332, #1546, #2014 ) ;
#4110=CARTESIAN_POINT ( 'NONE',  ( -365.9639710083354203, 1.530808498934204340E-15, 196.9298978568966163 ) ) ;
#4111=DIRECTION ( 'NONE',  ( -0.09383933793885568253, 2.673190762809473730E-31, 0.9955873536034882676 ) ) ;
#4112=ORIENTED_EDGE ( 'NONE', *, *, #1653, .T. ) ;
#4118=CIRCLE ( 'NONE', #1730, 30.50000000000113332 ) ;
#4123=CARTESIAN_POINT ( 'NONE',  ( 11.65031622824785984, 2.276824562219551028E-15, 35.95348720223918804 ) ) ;
#4124=LINE ( 'NONE', #353, #4349 ) ;
#4126=CARTESIAN_POINT ( 'NONE',  ( -57.28677601057306390, 25.00000000000018474, 546.4981013186294376 ) ) ;
#4127=CARTESIAN_POINT ( 'NONE',  ( -72.60637664584184847, 3.252606517456513302E-16, 552.9197695054128872 ) ) ;
#4129=VERTEX_POINT ( 'NONE', #2131 ) ;
#4130=CARTESIAN_POINT ( 'NONE',  ( -48.20943979673047863, 3.740497495074990297E-15, 509.2978244404888528 ) ) ;
#4132=EDGE_CURVE ( 'NONE', #8, #2651, #3809, .T. ) ;
#4137=ORIENTED_EDGE ( 'NONE', *, *, #3088, .T. ) ;
#4138=EDGE_LOOP ( 'NONE', ( #636, #4762 ) ) ;
#4143=AXIS2_PLACEMENT_3D ( 'NONE', #908, #2174, #958 ) ;
#4144=AXIS2_PLACEMENT_3D ( 'NONE', #2113, #4670, #2556 ) ;
#4150=FACE_OUTER_BOUND ( 'NONE', #4058, .T. ) ;
#4153=CARTESIAN_POINT ( 'NONE',  ( 4.992201166475890517, 1.572093150103981429E-15, 252.6216919286947586 ) ) ;
#4154=CARTESIAN_POINT ( 'NONE',  ( -12.39202333278750601, 25.00000000000000355, 98.84296066633362443 ) ) ;
#4155=CARTESIAN_POINT ( 'NONE',  ( -1.533280346156490337, 2.222614453595284090E-15, 488.4857301958385278 ) ) ;
#4157=ORIENTED_EDGE ( 'NONE', *, *, #4298, .F. ) ;
#4159=DIRECTION ( 'NONE',  ( -0.01527226085271972227, -2.080004339938201146E-31, -0.9998833722232041143 ) ) ;
#4160=ADVANCED_FACE ( 'NONE', ( #4795 ), #1470, .T. ) ;
#4161=( NAMED_UNIT ( * ) SI_UNIT ( $, .STERADIAN. ) SOLID_ANGLE_UNIT ( ) );
#4163=TOROIDAL_SURFACE ( 'NONE', #1782, 28.50000000000115463, 1.000000000000000000 ) ;
#4164=ORIENTED_EDGE ( 'NONE', *, *, #4230, .F. ) ;
#4165=EDGE_LOOP ( 'NONE', ( #4047, #5116 ) ) ;
#4174=ORIENTED_EDGE ( 'NONE', *, *, #3662, .T. ) ;
#4175=AXIS2_PLACEMENT_3D ( 'NONE', #3747, #1593, #2038 ) ;
#4176=DIRECTION ( 'NONE',  ( 0.09383933793885568253, -2.673190762809473730E-31, -0.9955873536034882676 ) ) ;
#4178=FACE_OUTER_BOUND ( 'NONE', #525, .T. ) ;
#4182=CARTESIAN_POINT ( 'NONE',  ( -0.4023372602957597799, 1.572093150103981429E-15, 421.4664991284013809 ) ) ;
#4183=CARTESIAN_POINT ( 'NONE',  ( -0.4023372603089575006, -24.99999999999981881, 421.4664991283988229 ) ) ;
#4189=ORIENTED_EDGE ( 'NONE', *, *, #1033, .F. ) ;
#4191=DIRECTION ( 'NONE',  ( -0.09383933793885537722, 2.626968444144180508E-31, 0.9955873536034883786 ) ) ;
#4192=FACE_BOUND ( 'NONE', #5196, .T. ) ;
#4194=AXIS2_PLACEMENT_3D ( 'NONE', #3503, #1812, #1894 ) ;
#4197=ORIENTED_EDGE ( 'NONE', *, *, #765, .T. ) ;
#4201=DIRECTION ( 'NONE',  ( -0.09383933793885537722, 2.611561004589082621E-31, 0.9955873536034883786 ) ) ;
#4202=DIRECTION ( 'NONE',  ( -0.9955873536034884896, 5.273458392682100368E-31, -0.09383933793885443353 ) ) ;
#4204=AXIS2_PLACEMENT_3D ( 'NONE', #1811, #2033, #4586 ) ;
#4206=CARTESIAN_POINT ( 'NONE',  ( -35.15684241565268309, -24.99999999999981881, 493.9702760599490716 ) ) ;
#4207=FACE_OUTER_BOUND ( 'NONE', #2634, .T. ) ;
#4208=ORIENTED_EDGE ( 'NONE', *, *, #1156, .F. ) ;
#4209=DIRECTION ( 'NONE',  ( -0.9955873536034882676, 5.406119142139367196E-31, -0.09383933793885596009 ) ) ;
#4212=VERTEX_POINT ( 'NONE', #2708 ) ;
#4220=CIRCLE ( 'NONE', #3955, 31.50000000000120082 ) ;
#4223=CARTESIAN_POINT ( 'NONE',  ( -338.5986743560152377, 14.95948628165116823, 39.80450035817695209 ) ) ;
#4225=CIRCLE ( 'NONE', #4143, 4.382543221487789076 ) ;
#4226=EDGE_CURVE ( 'NONE', #3842, #463, #488, .T. ) ;
#4227=DIRECTION ( 'NONE',  ( 0.9955873536034882676, -5.475514420260265162E-31, 0.09383933793885552987 ) ) ;
#4230=EDGE_CURVE ( 'NONE', #342, #860, #2750, .T. ) ;
#4231=DIRECTION ( 'NONE',  ( 0.09383933793885537722, -2.626968444144180508E-31, -0.9955873536034883786 ) ) ;
#4232=CARTESIAN_POINT ( 'NONE',  ( 9.699276322990401766, -24.99999999999981881, 297.8714164406044915 ) ) ;
#4234=ORIENTED_EDGE ( 'NONE', *, *, #4132, .T. ) ;
#4235=TOROIDAL_SURFACE ( 'NONE', #2296, 23.00000000000115108, 2.000000000000000000 ) ;
#4237=FACE_OUTER_BOUND ( 'NONE', #3713, .T. ) ;
#4240=EDGE_LOOP ( 'NONE', ( #523, #4251 ) ) ;
#4242=DIRECTION ( 'NONE',  ( 0.09383933793885568253, -2.673190762809473730E-31, -0.9955873536034882676 ) ) ;
#4243=CARTESIAN_POINT ( 'NONE',  ( -52.92425795463013571, -24.99999999999981881, 513.6488213284161475 ) ) ;
#4244=CIRCLE ( 'NONE', #291, 27.43532828739476415 ) ;
#4247=CIRCLE ( 'NONE', #470, 1.000000000000000888 ) ;
#4248=ORIENTED_EDGE ( 'NONE', *, *, #756, .F. ) ;
#4251=ORIENTED_EDGE ( 'NONE', *, *, #971, .T. ) ;
#4254=FACE_OUTER_BOUND ( 'NONE', #3359, .T. ) ;
#4255=CIRCLE ( 'NONE', #3112, 12.50000000000009237 ) ;
#4256=B_SPLINE_CURVE_WITH_KNOTS ( 'NONE', 3,
 ( #248, #4757, #1503, #1922, #4713, #4452, #3006, #1819, #4859, #2363, #4043, #581, #2645, #3880, #3200, #942, #2599, #3609, #554, #274, #3856, #88, #4274, #1356, #4302, #3041, #2239, #504, #3512, #2625, #969, #1410, #997, #2211, #528, #3637, #2185, #115 ),
 .UNSPECIFIED., .F., .F.,
 ( 4, 2, 2, 2, 2, 2, 2, 2, 2, 2, 2, 2, 2, 2, 2, 2, 2, 2, 4 ),
 ( 0.000000000000000000, 0.1028767157186024211, 0.2057534314372048423, 0.2571917892965060459, 0.3086301471558072773, 0.3600685050151084532, 0.4115068628744096846, 0.4558387458985032614, 0.4780046874105500776, 0.5001706289225968938, 0.5231687412733679876, 0.5461668536241390814, 0.5921630783256812691, 0.6381593030272234568, 0.6841555277287657555, 0.7631166457965743444, 0.8420777638643828222, 0.9210388819321914111, 1.000000000000000000 ),
 .UNSPECIFIED. ) ;
#4258=DIRECTION ( 'NONE',  ( 0.9955873536034882676, -5.498835694391114214E-31, 0.09383933793885514130 ) ) ;
#4259=ORIENTED_EDGE ( 'NONE', *, *, #4654, .F. ) ;
#4260=TOROIDAL_SURFACE ( 'NONE', #2420, 28.50000000000115818, 1.000000000000000000 ) ;
#4261=AXIS2_PLACEMENT_3D ( 'NONE', #2522, #2099, #1634 ) ;
#4262=CARTESIAN_POINT ( 'NONE',  ( -48.20943979673047863, 3.740497495074990297E-15, 509.2978244404888528 ) ) ;
#4263=CARTESIAN_POINT ( 'NONE',  ( 8.821273309634928950, -24.99999999999981881, 380.5076279642381110 ) ) ;
#4266=ORIENTED_EDGE ( 'NONE', *, *, #1465, .F. ) ;
#4267=EDGE_CURVE ( 'NONE', #4320, #276, #2861, .T. ) ;
#4268=ORIENTED_EDGE ( 'NONE', *, *, #798, .F. ) ;
#4269=DIRECTION ( 'NONE',  ( 0.09383933793885568253, -2.673190762809473730E-31, -0.9955873536034882676 ) ) ;
#4270=ORIENTED_EDGE ( 'NONE', *, *, #5188, .T. ) ;
#4273=CARTESIAN_POINT ( 'NONE',  ( 11.35554381054933160, -24.99999999999981881, 353.5846600851155017 ) ) ;
#4274=CARTESIAN_POINT ( 'NONE',  ( -80.60298687151650654, 2.222614453595284090E-15, 555.2885198911399129 ) ) ;
#4275=DIRECTION ( 'NONE',  ( 0.09383933793885568253, -2.673190762809473730E-31, -0.9955873536034882676 ) ) ;
#4276=EDGE_LOOP ( 'NONE', ( #257, #3046, #4579, #507 ) ) ;
#4277=VERTEX_POINT ( 'NONE', #3493 ) ;
#4278=ORIENTED_EDGE ( 'NONE', *, *, #5358, .F. ) ;
#4279=DIRECTION ( 'NONE',  ( 0.09383933793885568253, -2.673190762809473730E-31, -0.9955873536034882676 ) ) ;
#4283=EDGE_LOOP ( 'NONE', ( #5248, #3712, #4590, #1361 ) ) ;
#4286=CARTESIAN_POINT ( 'NONE',  ( -5.157059352427092236, -24.99999999999981881, 435.5986320196304860 ) ) ;
#4287=DIRECTION ( 'NONE',  ( -0.09383933793885537722, 2.626968444144180508E-31, 0.9955873536034883786 ) ) ;
#4292=LINE ( 'NONE', #415, #4312 ) ;
#4296=CARTESIAN_POINT ( 'NONE',  ( -36.58361131987991399, 0.000000000000000000, 532.6725316595221784 ) ) ;
#4297=VERTEX_POINT ( 'NONE', #950 ) ;
#4298=EDGE_CURVE ( 'NONE', #936, #2195, #1052, .T. ) ;
#4299=EDGE_CURVE ( 'NONE', #4129, #911, #3049, .T. ) ;
#4301=CARTESIAN_POINT ( 'NONE',  ( -268.5984117390373171, -25.00000000000003197, 475.6392848759601293 ) ) ;
#4302=CARTESIAN_POINT ( 'NONE',  ( -122.4270646331731598, 3.252606517456513302E-16, 560.5113017241549187 ) ) ;
#4303=DIRECTION ( 'NONE',  ( -0.9955873536034883786, 5.430490990731020552E-31, -0.09383933793885548824 ) ) ;
#4305=ORIENTED_EDGE ( 'NONE', *, *, #3890, .T. ) ;
#4306=VERTEX_POINT ( 'NONE', #4385 ) ;
#4307=VERTEX_POINT ( 'NONE', #288 ) ;
#4308=DIRECTION ( 'NONE',  ( -0.09383933793885568253, 2.673190762809473730E-31, 0.9955873536034882676 ) ) ;
#4309=DIRECTION ( 'NONE',  ( -0.9955873536034882676, 5.452307672560250687E-31, -0.09383933793885569641 ) ) ;
#4311=ORIENTED_EDGE ( 'NONE', *, *, #4862, .F. ) ;
#4312=VECTOR ( 'NONE', #521, 1000.000000000000114 ) ;
#4313=CARTESIAN_POINT ( 'NONE',  ( -338.5048350180761076, 2.276824562219559311E-15, 38.80891300457378890 ) ) ;
#4314=CARTESIAN_POINT ( 'NONE',  ( -354.3266237013165778, -24.99999999999981881, 381.2801272015587983 ) ) ;
#4316=EDGE_CURVE ( 'NONE', #276, #4320, #2576, .T. ) ;
#4317=DIRECTION ( 'NONE',  ( -0.9955873536034882676, 5.452307672560245432E-31, -0.09383933793885568253 ) ) ;
#4318=CARTESIAN_POINT ( 'NONE',  ( -341.0742871682481905, -6.873162489031925530E-30, 199.2758813053679887 ) ) ;
#4320=VERTEX_POINT ( 'NONE', #5366 ) ;
#4321=CARTESIAN_POINT ( 'NONE',  ( 29.77542608467487995, 25.00000000000000355, 249.2409987768023711 ) ) ;
#4324=CIRCLE ( 'NONE', #984, 27.50000000000126477 ) ;
#4326=DIRECTION ( 'NONE',  ( -1.000000000000000000, -1.219242865862094703E-16, 0.000000000000000000 ) ) ;
#4328=CIRCLE ( 'NONE', #104, 1.000000000000000888 ) ;
#4329=VERTEX_POINT ( 'NONE', #1995 ) ;
#4331=VERTEX_POINT ( 'NONE', #236 ) ;
#4332=CARTESIAN_POINT ( 'NONE',  ( -338.5986743560152377, 14.95948628165116823, 39.80450035817695209 ) ) ;
#4333=DIRECTION ( 'NONE',  ( 0.09383933793885537722, -2.626968444144180508E-31, -0.9955873536034883786 ) ) ;
#4334=CARTESIAN_POINT ( 'NONE',  ( -353.5191290882918338, 0.000000000000000000, 198.1028895811323025 ) ) ;
#4336=EDGE_LOOP ( 'NONE', ( #1763, #3937, #1623, #2786 ) ) ;
#4339=CARTESIAN_POINT ( 'NONE',  ( -30.63277980166695258, 0.000000000000000000, 527.1358351633697339 ) ) ;
#4341=AXIS2_PLACEMENT_3D ( 'NONE', #3220, #3704, #4413 ) ;
#4343=CIRCLE ( 'NONE', #4951, 4.382543221487789964 ) ;
#4344=AXIS2_PLACEMENT_3D ( 'NONE', #3303, #70, #1305 ) ;
#4345=AXIS2_PLACEMENT_3D ( 'NONE', #1670, #4191, #1270 ) ;
#4347=CARTESIAN_POINT ( 'NONE',  ( -367.0460729392618759, 0.000000000000000000, 268.0688838304710089 ) ) ;
#4348=( NAMED_UNIT ( * ) SI_UNIT ( $, .STERADIAN. ) SOLID_ANGLE_UNIT ( ) );
#4349=VECTOR ( 'NONE', #1915, 1000.000000000000000 ) ;
#4351=CARTESIAN_POINT ( 'NONE',  ( 5.624351423727398824, 25.00000000000018474, 474.0483466084681368 ) ) ;
#4355=DIRECTION ( 'NONE',  ( -0.09383933793885568253, 2.673190762809473730E-31, 0.9955873536034882676 ) ) ;
#4356=FACE_BOUND ( 'NONE', #1847, .T. ) ;
#4358=EDGE_LOOP ( 'NONE', ( #119, #4730, #633, #3824 ) ) ;
#4360=DIRECTION ( 'NONE',  ( -0.09383933793885568253, 2.673190762809473730E-31, 0.9955873536034882676 ) ) ;
#4367=CARTESIAN_POINT ( 'NONE',  ( 34.60640066538633874, 2.222614453595284090E-15, 295.6817845355787995 ) ) ;
#4371=CARTESIAN_POINT ( 'NONE',  ( 35.78913469918393275, 25.00000000000018474, 310.6402212931347435 ) ) ;
#4373=AXIS2_PLACEMENT_3D ( 'NONE', #3180, #2404, #4407 ) ;
#4376=CARTESIAN_POINT ( 'NONE',  ( 5.624351423727524946, 2.222614453595284090E-15, 474.0483466084679662 ) ) ;
#4380=EDGE_CURVE ( 'NONE', #281, #2877, #117, .T. ) ;
#4381=EDGE_LOOP ( 'NONE', ( #2455, #2164, #1627, #5163 ) ) ;
#4384=DIRECTION ( 'NONE',  ( -0.01527226085271972227, -2.080004339938201146E-31, -0.9998833722232041143 ) ) ;
#4385=CARTESIAN_POINT ( 'NONE',  ( -323.1537148033839344, 3.735172737399554547E-15, 200.9649893882672984 ) ) ;
#4389=ADVANCED_FACE ( 'NONE', ( #4031 ), #1578, .F. ) ;
#4390=CARTESIAN_POINT ( 'NONE',  ( -367.0882437885064746, -24.99999999999981881, 297.8351940652706276 ) ) ;
#4394=FACE_OUTER_BOUND ( 'NONE', #4739, .T. ) ;
#4395=CARTESIAN_POINT ( 'NONE',  ( 33.59898979596731294, 5.421010862427522170E-17, 384.0431050523496310 ) ) ;
#4396=CARTESIAN_POINT ( 'NONE',  ( 10.82492224058160879, -24.99999999999981881, 312.2165827548579387 ) ) ;
#4398=ORIENTED_EDGE ( 'NONE', *, *, #4860, .F. ) ;
#4399=CARTESIAN_POINT ( 'NONE',  ( -86.97194166595193110, 25.00000000000018474, 531.0655262460722952 ) ) ;
#4402=( LENGTH_UNIT ( ) NAMED_UNIT ( * ) SI_UNIT ( .MILLI., .METRE. ) );
#4403=VERTEX_POINT ( 'NONE', #3268 ) ;
#4405=DIRECTION ( 'NONE',  ( -0.09383933793885537722, 2.626968444144180508E-31, 0.9955873536034883786 ) ) ;
#4407=DIRECTION ( 'NONE',  ( -0.9955873536034882676, 5.452307672560245432E-31, -0.09383933793885568253 ) ) ;
#4413=DIRECTION ( 'NONE',  ( -0.9955873536034882676, 5.452307672560245432E-31, -0.09383933793885568253 ) ) ;
#4414=CARTESIAN_POINT ( 'NONE',  ( -80.60298687151718866, -24.99999999999981881, 555.2885198911441194 ) ) ;
#4417=CIRCLE ( 'NONE', #2049, 31.50000000000125766 ) ;
#4419=AXIS2_PLACEMENT_3D ( 'NONE', #4767, #537, #1805 ) ;
#4421=DIRECTION ( 'NONE',  ( -1.219242865862094703E-16, 1.000000000000000000, -1.149200448409285278E-17 ) ) ;
#4422=CARTESIAN_POINT ( 'NONE',  ( -207.8397519515728504, 5.421010862427522170E-17, 541.5412455041541762 ) ) ;
#4424=CARTESIAN_POINT ( 'NONE',  ( 36.66581985038887126, -24.99999999999981881, 340.1662229844756098 ) ) ;
#4427=CARTESIAN_POINT ( 'NONE',  ( -5.157059352426552223, 3.740497495074990297E-15, 435.5986320196309975 ) ) ;
#4433=CIRCLE ( 'NONE', #2063, 21.00000000000124700 ) ;
#4435=VERTEX_POINT ( 'NONE', #4493 ) ;
#4438=CARTESIAN_POINT ( 'NONE',  ( -0.6802310551622114954, 2.222614453595284090E-15, 47.14310755735262859 ) ) ;
#4439=FACE_OUTER_BOUND ( 'NONE', #3930, .T. ) ;
#4442=ORIENTED_EDGE ( 'NONE', *, *, #224, .T. ) ;
#4444=CYLINDRICAL_SURFACE ( 'NONE', #5151, 4.382543221487789964 ) ;
#4445=CYLINDRICAL_SURFACE ( 'NONE', #1243, 31.50000000000114397 ) ;
#4448=CARTESIAN_POINT ( 'NONE',  ( -346.0119820531829191, 0.000000000000000000, 118.4559012928527721 ) ) ;
#4449=CARTESIAN_POINT ( 'NONE',  ( -0.4023372602832280820, 25.00000000000018474, 421.4664991283991640 ) ) ;
#4451=CARTESIAN_POINT ( 'NONE',  ( -122.4270646331732451, -24.99999999999981881, 560.5113017241552598 ) ) ;
#4452=CARTESIAN_POINT ( 'NONE',  ( 34.60640066538633874, 2.222614453595284090E-15, 295.6817845355787995 ) ) ;
#4454=CARTESIAN_POINT ( 'NONE',  ( -174.3534642324312358, 25.00000000000018474, 552.7876087698487027 ) ) ;
#4455=ORIENTED_EDGE ( 'NONE', *, *, #111, .F. ) ;
#4458=CARTESIAN_POINT ( 'NONE',  ( -372.5496767551892958, 2.625968386833887277E-15, 176.2205164123462282 ) ) ;
#4460=EDGE_CURVE ( 'NONE', #249, #3236, #24, .T. ) ;
#4461=CLOSED_SHELL ( 'NONE', ( #3500, #1717, #3727, #882 ) ) ;
#4466=DIRECTION ( 'NONE',  ( -1.000000000000000000, -1.219242865862094703E-16, 0.000000000000000000 ) ) ;
#4470=CARTESIAN_POINT ( 'NONE',  ( -334.2354697480813002, 14.95948628165116823, 40.21575531256979019 ) ) ;
#4471=ORIENTED_EDGE ( 'NONE', *, *, #4096, .F. ) ;
#4474=DIRECTION ( 'NONE',  ( -0.09383933793885568253, 2.673190762809473730E-31, 0.9955873536034882676 ) ) ;
#4476=LINE ( 'NONE', #4802, #196 ) ;
#4477=CARTESIAN_POINT ( 'NONE',  ( -351.6423423295148041, 5.421010862427522170E-17, 178.1911425090623311 ) ) ;
#4478=CARTESIAN_POINT ( 'NONE',  ( -48.20943979671786650, 25.00000000000018474, 509.2978244404892507 ) ) ;
#4479=CARTESIAN_POINT ( 'NONE',  ( -36.58361131987991399, 0.000000000000000000, 532.6725316595221784 ) ) ;
#4482=CARTESIAN_POINT ( 'NONE',  ( -12.39202333278749357, 1.572093150103981429E-15, 98.84296066633379496 ) ) ;
#4483=AXIS2_PLACEMENT_3D ( 'NONE', #5364, #2044, #398 ) ;
#4487=ADVANCED_FACE ( 'NONE', ( #1520 ), #694, .T. ) ;
#4492=CARTESIAN_POINT ( 'NONE',  ( -349.7655555707380017, 2.222614453595284090E-15, 158.2793954369929850 ) ) ;
#4493=CARTESIAN_POINT ( 'NONE',  ( -321.3913159930368693, 5.712857831165385696E-15, 160.9538165682496640 ) ) ;
#4494=DIRECTION ( 'NONE',  ( -0.9955873536034882676, 0.000000000000000000, -0.09383933793885600172 ) ) ;
#4495=ORIENTED_EDGE ( 'NONE', *, *, #3821, .F. ) ;
#4496=FACE_OUTER_BOUND ( 'NONE', #1466, .T. ) ;
#4497=CARTESIAN_POINT ( 'NONE',  ( -334.2906958041416488, 0.000000000000000000, 430.9840019716568804 ) ) ;
#4498=DIRECTION ( 'NONE',  ( 0.09383933793885537722, -2.626968444144180508E-31, -0.9955873536034883786 ) ) ;
#4502=CARTESIAN_POINT ( 'NONE',  ( -23.53079058812344471, 25.00000000000018474, 476.4235034963351154 ) ) ;
#4503=CARTESIAN_POINT ( 'NONE',  ( -364.1439395362590403, -24.99999999999981881, 237.2787335496889227 ) ) ;
#4504=AXIS2_PLACEMENT_3D ( 'NONE', #709, #1188, #2396 ) ;
#4509=CARTESIAN_POINT ( 'NONE',  ( -213.0979982360508416, 24.99999999999997158, 511.7519955242232754 ) ) ;
#4513=( GEOMETRIC_REPRESENTATION_CONTEXT ( 3 ) GLOBAL_UNCERTAINTY_ASSIGNED_CONTEXT ( ( #3094 ) ) GLOBAL_UNIT_ASSIGNED_CONTEXT ( ( #852, #5387, #4161 ) ) REPRESENTATION_CONTEXT ( 'NONE', 'WORKASPACE' ) );
#4522=CARTESIAN_POINT ( 'NONE',  ( -340.0535087002904220, -14.95948628165117178, 101.9421712359864500 ) ) ;
#4525=AXIS2_PLACEMENT_3D ( 'NONE', #4334, #3461, #1826 ) ;
#4530=DIRECTION ( 'NONE',  ( -0.9955873536034884896, 5.452307672560235798E-31, -0.09383933793885443353 ) ) ;
#4531=DIRECTION ( 'NONE',  ( -0.09383933793885537722, 2.626968444144180508E-31, 0.9955873536034883786 ) ) ;
#4533=EDGE_CURVE ( 'NONE', #1814, #2651, #4247, .T. ) ;
#4539=CARTESIAN_POINT ( 'NONE',  ( -354.3266237013165778, 25.00000000000018474, 381.2801272015587983 ) ) ;
#4540=CARTESIAN_POINT ( 'NONE',  ( -285.5643670724598451, 2.222614453595284090E-15, 494.2304181244439292 ) ) ;
#4542=CARTESIAN_POINT ( 'NONE',  ( -16.96312831416352296, 1.572093150103981429E-15, 463.2830513152439380 ) ) ;
#4544=DIRECTION ( 'NONE',  ( -0.09383933793885537722, 2.626968444144180508E-31, 0.9955873536034883786 ) ) ;
#4545=CARTESIAN_POINT ( 'NONE',  ( -349.6717162327985307, 3.252606517456513302E-16, 157.2838080833889194 ) ) ;
#4547=AXIS2_PLACEMENT_3D ( 'NONE', #2730, #2442, #4530 ) ;
#4549=DIRECTION ( 'NONE',  ( -0.09383933793885536334, 2.626968444144180070E-31, 0.9955873536034882676 ) ) ;
#4555=EDGE_CURVE ( 'NONE', #861, #3068, #385, .T. ) ;
#4556=CARTESIAN_POINT ( 'NONE',  ( -353.4921497144319460, 2.222614453595284090E-15, 38.40071206960160310 ) ) ;
#4557=ORIENTED_EDGE ( 'NONE', *, *, #3893, .F. ) ;
#4558=ORIENTED_EDGE ( 'NONE', *, *, #2515, .T. ) ;
#4560=DIRECTION ( 'NONE',  ( -0.9955873536034882676, 5.484003909441380272E-31, -0.09383933793885536334 ) ) ;
#4563=ADVANCED_FACE ( 'NONE', ( #5418, #3321 ), #1272, .F. ) ;
#4564=CARTESIAN_POINT ( 'NONE',  ( -349.8593949086763928, 2.222614453595284090E-15, 159.2749827905956010 ) ) ;
#4565=CARTESIAN_POINT ( 'NONE',  ( 4.992201166475765284, 25.00000000000018474, 252.6216919286950429 ) ) ;
#4566=CARTESIAN_POINT ( 'NONE',  ( -105.2090356704102447, -24.99999999999981881, 560.1816718768288865 ) ) ;
#4567=EDGE_CURVE ( 'NONE', #1142, #1648, #3467, .T. ) ;
#4568=VERTEX_POINT ( 'NONE', #370 ) ;
#4571=CARTESIAN_POINT ( 'NONE',  ( -13.34676807733242754, 3.807633061153780218E-15, 36.33529372355719289 ) ) ;
#4574=CARTESIAN_POINT ( 'NONE',  ( -375.4961969329172575, 3.911847525938617771E-15, 95.58821507570917220 ) ) ;
#4576=DIRECTION ( 'NONE',  ( 0.01527226085271972227, 2.095411779493299033E-31, 0.9998833722232041143 ) ) ;
#4579=ORIENTED_EDGE ( 'NONE', *, *, #4057, .T. ) ;
#4580=DIRECTION ( 'NONE',  ( -0.09383933793885537722, 2.626968444144180508E-31, 0.9955873536034883786 ) ) ;
#4582=PLANE ( 'NONE',  #3478 ) ;
#4583=ADVANCED_FACE ( 'NONE', ( #5004 ), #3797, .F. ) ;
#4585=AXIS2_PLACEMENT_3D ( 'NONE', #4766, #1804, #5149 ) ;
#4586=DIRECTION ( 'NONE',  ( -0.9955873536034882676, 5.273458392682099492E-31, -0.09383933793885600172 ) ) ;
#4587=CARTESIAN_POINT ( 'NONE',  ( 11.65205807320727871, -24.99999999999981881, 340.0738060255407049 ) ) ;
#4589=AXIS2_PLACEMENT_3D ( 'NONE', #4922, #1109, #1519 ) ;
#4590=ORIENTED_EDGE ( 'NONE', *, *, #3629, .T. ) ;
#4597=ADVANCED_FACE ( 'NONE', ( #859 ), #2046, .T. ) ;
#4599=CARTESIAN_POINT ( 'NONE',  ( -317.6377424754826393, 3.490243377570163137E-15, 121.1303224241101049 ) ) ;
#4602=CARTESIAN_POINT ( 'NONE',  ( -0.8482259245422840710, 2.276824562219559311E-15, 36.14439046289818691 ) ) ;
#4604=AXIS2_PLACEMENT_3D ( 'NONE', #487, #4580, #809 ) ;
#4605=ORIENTED_EDGE ( 'NONE', *, *, #4555, .F. ) ;
#4610=FACE_OUTER_BOUND ( 'NONE', #3961, .T. ) ;
#4611=CIRCLE ( 'NONE', #4696, 1.000000000000000888 ) ;
#4612=CARTESIAN_POINT ( 'NONE',  ( -213.0979982360508416, -25.00000000000003197, 511.7519955242232754 ) ) ;
#4613=CARTESIAN_POINT ( 'NONE',  ( -336.1069982926118769, 1.517883041479706208E-15, 349.6877309229317916 ) ) ;
#4614=CARTESIAN_POINT ( 'NONE',  ( -312.0566616799237067, 1.517883041479706208E-15, 419.2731246273846182 ) ) ;
#4617=VERTEX_POINT ( 'NONE', #2517 ) ;
#4618=FACE_OUTER_BOUND ( 'NONE', #722, .T. ) ;
#4621=AXIS2_PLACEMENT_3D ( 'NONE', #2456, #4159, #3234 ) ;
#4622=ORIENTED_EDGE ( 'NONE', *, *, #869, .T. ) ;
#4627=CARTESIAN_POINT ( 'NONE',  ( -353.5191290882918338, 0.000000000000000000, 198.1028895811327573 ) ) ;
#4628=DIRECTION ( 'NONE',  ( -5.679099018122554920E-31, -1.000000000000000000, 2.149753974990777610E-31 ) ) ;
#4632=ORIENTED_EDGE ( 'NONE', *, *, #3355, .F. ) ;
#4633=EDGE_LOOP ( 'NONE', ( #1362, #600, #4051, #888 ) ) ;
#4634=EDGE_LOOP ( 'NONE', ( #2839, #4234, #2324, #4268 ) ) ;
#4636=CARTESIAN_POINT ( 'NONE',  ( -334.2354697480813002, -14.95948628165117178, 40.21575531256979019 ) ) ;
#4639=CARTESIAN_POINT ( 'NONE',  ( -16.96312831416352296, 1.572093150103981429E-15, 463.2830513152439380 ) ) ;
#4640=CARTESIAN_POINT ( 'NONE',  ( -152.2642418386349163, 3.740497495074990297E-15, 532.1805559224781064 ) ) ;
#4642=CIRCLE ( 'NONE', #3249, 31.50000000000114397 ) ;
#4644=VERTEX_POINT ( 'NONE', #1761 ) ;
#4646=CARTESIAN_POINT ( 'NONE',  ( 0.000000000000000000, 0.000000000000000000, 0.000000000000000000 ) ) ;
#4647=DIRECTION ( 'NONE',  ( -0.9955873536034882676, 5.452307672560245432E-31, -0.09383933793885568253 ) ) ;
#4649=DIRECTION ( 'NONE',  ( -0.09383933793885568253, 2.673190762809473730E-31, 0.9955873536034882676 ) ) ;
#4652=CARTESIAN_POINT ( 'NONE',  ( -357.2727026058461206, 5.421010862427522170E-17, 237.9263837252718758 ) ) ;
#4654=EDGE_CURVE ( 'NONE', #4403, #2695, #5291, .T. ) ;
#4655=DIRECTION ( 'NONE',  ( -5.720779902258401340E-31, -1.000000000000000000, 2.099398147291833041E-31 ) ) ;
#4656=ORIENTED_EDGE ( 'NONE', *, *, #5089, .F. ) ;
#4660=DIRECTION ( 'NONE',  ( -0.9955873536034882676, 5.498529991225541720E-31, -0.09383933793885536334 ) ) ;
#4662=( NAMED_UNIT ( * ) SI_UNIT ( $, .STERADIAN. ) SOLID_ANGLE_UNIT ( ) );
#4664=CARTESIAN_POINT ( 'NONE',  ( -342.0170653153606395, 3.740497495074990297E-15, 268.9367132353195302 ) ) ;
#4665=CARTESIAN_POINT ( 'NONE',  ( -342.0170653153606395, 3.740497495074990297E-15, 268.9367132353195302 ) ) ;
#4669=VERTEX_POINT ( 'NONE', #2212 ) ;
#4670=DIRECTION ( 'NONE',  ( 0.09383933793885568253, -2.673190762809473730E-31, -0.9955873536034882676 ) ) ;
#4673=CIRCLE ( 'NONE', #194, 12.50000000000002842 ) ;
#4675=DIRECTION ( 'NONE',  ( 1.000000000000000000, -3.851859888774468203E-31, 0.000000000000000000 ) ) ;
#4677=CARTESIAN_POINT ( 'NONE',  ( -8.629236981504860182, -25.00000000000000355, 142.6115645898824198 ) ) ;
#4678=CIRCLE ( 'NONE', #3366, 12.50000000000009237 ) ;
#4682=FACE_OUTER_BOUND ( 'NONE', #5345, .T. ) ;
#4687=ORIENTED_EDGE ( 'NONE', *, *, #2496, .T. ) ;
#4689=DIRECTION ( 'NONE',  ( 0.09383933793885568253, -2.673190762809473730E-31, -0.9955873536034882676 ) ) ;
#4692=CARTESIAN_POINT ( 'NONE',  ( -353.5191290882918338, 0.000000000000000000, 198.1028895811323025 ) ) ;
#4695=CIRCLE ( 'NONE', #3995, 21.00000000000124700 ) ;
#4696=AXIS2_PLACEMENT_3D ( 'NONE', #1247, #3806, #5422 ) ;
#4697=DIRECTION ( 'NONE',  ( -0.9955873536034884896, 5.462637660443545995E-31, -0.09383933793885503027 ) ) ;
#4699=CARTESIAN_POINT ( 'NONE',  ( -152.2642418387488874, -24.99999999999981881, 532.1805559224803801 ) ) ;
#4700=CARTESIAN_POINT ( 'NONE',  ( -344.4167133082243595, -14.95948628165117178, 101.5309162815936048 ) ) ;
#4705=VERTEX_POINT ( 'NONE', #3857 ) ;
#4709=CARTESIAN_POINT ( 'NONE',  ( -1.533280346156490337, 2.222614453595284090E-15, 488.4857301958385278 ) ) ;
#4712=CARTESIAN_POINT ( 'NONE',  ( -121.8424039465433566, -24.99999999999981881, 535.4314447305355316 ) ) ;
#4713=CARTESIAN_POINT ( 'NONE',  ( 29.77542608467492613, 2.222614453595284090E-15, 249.2409987768030533 ) ) ;
#4715=ORIENTED_EDGE ( 'NONE', *, *, #4855, .F. ) ;
#4716=ORIENTED_EDGE ( 'NONE', *, *, #2102, .F. ) ;
#4719=CARTESIAN_POINT ( 'NONE',  ( -338.5986743560152377, 14.95948628165116823, 39.80450035817695209 ) ) ;
#4721=CARTESIAN_POINT ( 'NONE',  ( -342.9618789639491752, 14.95948628165116823, 39.39324540378412109 ) ) ;
#4722=PLANE ( 'NONE',  #2140 ) ;
#4724=TOROIDAL_SURFACE ( 'NONE', #2443, 30.50000000000110845, 1.000000000000000000 ) ;
#4725=CARTESIAN_POINT ( 'NONE',  ( -323.2681027518141263, 5.712857831165387273E-15, 180.8655636403200333 ) ) ;
#4726=CARTESIAN_POINT ( 'NONE',  ( -342.0170653153610374, -24.99999999999981881, 268.9367132353194734 ) ) ;
#4728=ADVANCED_FACE ( 'NONE', ( #1357 ), #1969, .F. ) ;
#4729=EDGE_CURVE ( 'NONE', #1390, #2722, #2500, .T. ) ;
#4730=ORIENTED_EDGE ( 'NONE', *, *, #4925, .F. ) ;
#4731=DIRECTION ( 'NONE',  ( 0.09383933793885568253, -2.673190762809473730E-31, -0.9955873536034882676 ) ) ;
#4732=FACE_BOUND ( 'NONE', #1867, .T. ) ;
#4733=EDGE_LOOP ( 'NONE', ( #5058, #4270, #3963, #1018 ) ) ;
#4734=CARTESIAN_POINT ( 'NONE',  ( 11.81831109762766729, 25.00000000000000355, 46.95220429669349471 ) ) ;
#4736=CARTESIAN_POINT ( 'NONE',  ( -249.5207023207451300, 1.843143693225357538E-15, 491.2832465756980014 ) ) ;
#4739=EDGE_LOOP ( 'NONE', ( #3922, #5362 ) ) ;
#4740=ORIENTED_EDGE ( 'NONE', *, *, #2457, .F. ) ;
#4741=EDGE_LOOP ( 'NONE', ( #4248, #2542, #4864, #1431 ) ) ;
#4742=FACE_BOUND ( 'NONE', #2508, .T. ) ;
#4745=AXIS2_PLACEMENT_3D ( 'NONE', #2071, #2921, #5 ) ;
#4747=CARTESIAN_POINT ( 'NONE',  ( -341.0742871682481905, -6.873162489031922727E-30, 199.2758813053679887 ) ) ;
#4748=CARTESIAN_POINT ( 'NONE',  ( -72.60637664584220374, -24.99999999999981881, 552.9197695054134556 ) ) ;
#4749=CARTESIAN_POINT ( 'NONE',  ( -375.4961969329172575, 3.911847525938617771E-15, 95.58821507570915799 ) ) ;
#4750=PLANE ( 'NONE',  #3762 ) ;
#4751=CARTESIAN_POINT ( 'NONE',  ( -354.3266237013149862, 5.421010862427522170E-17, 381.2801272015580025 ) ) ;
#4753=CARTESIAN_POINT ( 'NONE',  ( -174.3534642324304116, 5.421010862427522170E-17, 552.7876087698471110 ) ) ;
#4757=CARTESIAN_POINT ( 'NONE',  ( 12.58979647763672283, 2.222614453595284090E-15, 97.46177917736021357 ) ) ;
#4760=ADVANCED_FACE ( 'NONE', ( #4682 ), #5191, .T. ) ;
#4761=ADVANCED_FACE ( 'NONE', ( #2676, #4356 ), #1844, .F. ) ;
#4762=ORIENTED_EDGE ( 'NONE', *, *, #1403, .T. ) ;
#4766=CARTESIAN_POINT ( 'NONE',  ( -353.4252897503525332, 0.000000000000000000, 197.1073022275279243 ) ) ;
#4767=CARTESIAN_POINT ( 'NONE',  ( -357.2727026058461206, 5.421010862427522170E-17, 237.9263837252718758 ) ) ;
#4769=DIRECTION ( 'NONE',  ( -0.9955873536034884896, 0.000000000000000000, -0.09383933793885443353 ) ) ;
#4770=EDGE_LOOP ( 'NONE', ( #1986, #26, #2009, #561 ) ) ;
#4773=CIRCLE ( 'NONE', #476, 4.382543221487789964 ) ;
#4774=CARTESIAN_POINT ( 'NONE',  ( -174.3534642324312358, -24.99999999999981881, 552.7876087698487027 ) ) ;
#4775=CARTESIAN_POINT ( 'NONE',  ( -17.67824838295694434, 4.358724120770099429E-15, 47.40273599184887132 ) ) ;
#4776=AXIS2_PLACEMENT_3D ( 'NONE', #3001, #3243, #4675 ) ;
#4777=VECTOR ( 'NONE', #586, 1000.000000000000000 ) ;
#4778=STYLED_ITEM('',(#5451),#1285);
#4781=CARTESIAN_POINT ( 'NONE',  ( 35.78913469918423829, 0.000000000000000000, 310.6402212931345161 ) ) ;
#4783=AXIS2_PLACEMENT_3D ( 'NONE', #2080, #5009, #1332 ) ;
#4785=CARTESIAN_POINT ( 'NONE',  ( -49.96441683051492078, 25.00000000000018474, 542.4422122871054626 ) ) ;
#4791=ORIENTED_EDGE ( 'NONE', *, *, #462, .T. ) ;
#4792=DIRECTION ( 'NONE',  ( 0.09383933793885568253, -2.673190762809473730E-31, -0.9955873536034882676 ) ) ;
#4793=EDGE_CURVE ( 'NONE', #1648, #2973, #475, .T. ) ;
#4795=FACE_OUTER_BOUND ( 'NONE', #4000, .T. ) ;
#4799=FACE_OUTER_BOUND ( 'NONE', #283, .T. ) ;
#4800=CARTESIAN_POINT ( 'NONE',  ( -223.9642223310802649, -25.00000000000003197, 534.3227077390027944 ) ) ;
#4802=CARTESIAN_POINT ( 'NONE',  ( 11.65031622824785984, 2.276824562219551028E-15, 35.95348720223918804 ) ) ;
#4804=FACE_OUTER_BOUND ( 'NONE', #1217, .T. ) ;
#4806=CARTESIAN_POINT ( 'NONE',  ( 12.58979647763662513, 25.00000000000000355, 97.46177917735926144 ) ) ;
#4813=FACE_OUTER_BOUND ( 'NONE', #3149, .T. ) ;
#4814=PLANE ( 'NONE',  #4373 ) ;
#4815=CARTESIAN_POINT ( 'NONE',  ( -338.5986743560152377, -14.95948628165117178, 39.80450035817695209 ) ) ;
#4817=DIRECTION ( 'NONE',  ( 0.9955873536034884896, -5.462637660443545995E-31, 0.09383933793885503027 ) ) ;
#4821=CARTESIAN_POINT ( 'NONE',  ( -19.78983854945535725, -24.99999999999981881, 515.1268587725797943 ) ) ;
#4824=DIRECTION ( 'NONE',  ( 0.01527226085271972227, 2.095411779493299033E-31, 0.9998833722232041143 ) ) ;
#4826=CARTESIAN_POINT ( 'NONE',  ( -19.78983854945535725, 25.00000000000018474, 515.1268587725797943 ) ) ;
#4828=CARTESIAN_POINT ( 'NONE',  ( 35.78913469918393275, -24.99999999999981881, 310.6402212931347435 ) ) ;
#4829=EDGE_LOOP ( 'NONE', ( #2983, #38 ) ) ;
#4830=CARTESIAN_POINT ( 'NONE',  ( -152.2642418385221674, 25.00000000000018474, 532.1805559224801527 ) ) ;
#4831=VERTEX_POINT ( 'NONE', #280 ) ;
#4837=CIRCLE ( 'NONE', #3280, 1.000000000000000888 ) ;
#4839=CARTESIAN_POINT ( 'NONE',  ( -332.6117946626184221, -1.154691298157368797E-29, 200.0735156778482917 ) ) ;
#4845=APPLICATION_CONTEXT ( 'automotive_design' ) ;
#4855=EDGE_CURVE ( 'NONE', #4277, #860, #1130, .T. ) ;
#4857=CARTESIAN_POINT ( 'NONE',  ( -80.60298687151650654, 2.222614453595284090E-15, 555.2885198911399129 ) ) ;
#4858=CARTESIAN_POINT ( 'NONE',  ( -80.59222536594943165, -24.99999999999981881, 529.1597157429057461 ) ) ;
#4859=CARTESIAN_POINT ( 'NONE',  ( 36.35777514575885760, 2.222614453595284090E-15, 354.7349908125909792 ) ) ;
#4860=EDGE_CURVE ( 'NONE', #4985, #1728, #4255, .T. ) ;
#4862=EDGE_CURVE ( 'NONE', #5281, #5060, #1875, .T. ) ;
#4864=ORIENTED_EDGE ( 'NONE', *, *, #4533, .T. ) ;
#4865=CARTESIAN_POINT ( 'NONE',  ( -107.0991749147297014, 25.00000000000018474, 535.0680222229608489 ) ) ;
#4868=DIRECTION ( 'NONE',  ( -0.09383933793885536334, 2.626968444144180070E-31, 0.9955873536034882676 ) ) ;
#4869=AXIS2_PLACEMENT_3D ( 'NONE', #374, #4176, #5007 ) ;
#4873=CARTESIAN_POINT ( 'NONE',  ( -344.4167133082243595, 2.222614453595284090E-15, 101.5309162815936048 ) ) ;
#4874=CARTESIAN_POINT ( 'NONE',  ( -347.9826081498995336, 2.222614453595284090E-15, 139.3632357185260560 ) ) ;
#4877=ORIENTED_EDGE ( 'NONE', *, *, #2647, .F. ) ;
#4878=EDGE_CURVE ( 'NONE', #689, #3599, #2369, .T. ) ;
#4880=CARTESIAN_POINT ( 'NONE',  ( -223.9642223310785312, 5.421010862427522170E-17, 534.3227077389987016 ) ) ;
#4883=CYLINDRICAL_SURFACE ( 'NONE', #2187, 4.382543221487789964 ) ;
#4884=CARTESIAN_POINT ( 'NONE',  ( -249.5207023207449879, 24.99999999999997158, 491.2832465756976035 ) ) ;
#4886=CARTESIAN_POINT ( 'NONE',  ( 23.50217280488020677, 5.421010862427522170E-17, 428.9062724124374881 ) ) ;
#4887=LINE ( 'NONE', #1124, #2226 ) ;
#4889=CARTESIAN_POINT ( 'NONE',  ( -342.0244061588616091, 25.00000000000018474, 297.0039604601892620 ) ) ;
#4890=ORIENTED_EDGE ( 'NONE', *, *, #4230, .T. ) ;
#4891=CIRCLE ( 'NONE', #2529, 30.50000000000124345 ) ;
#4892=FACE_OUTER_BOUND ( 'NONE', #3422, .T. ) ;
#4895=UNCERTAINTY_MEASURE_WITH_UNIT (LENGTH_MEASURE( 1.000000000000000082E-05 ), #1289, 'distance_accuracy_value', 'NONE');
#4898=DIRECTION ( 'NONE',  ( 0.9955873536034882676, -5.273458392682099492E-31, 0.09383933793885600172 ) ) ;
#4900=DIRECTION ( 'NONE',  ( -0.9955873536034882676, 5.436595176548168253E-31, -0.09383933793885512742 ) ) ;
#4901=ORIENTED_EDGE ( 'NONE', *, *, #2982, .F. ) ;
#4904=FACE_OUTER_BOUND ( 'NONE', #2918, .T. ) ;
#4908=DIRECTION ( 'NONE',  ( -0.09383933793885537722, 2.626968444144180508E-31, 0.9955873536034883786 ) ) ;
#4909=CARTESIAN_POINT ( 'NONE',  ( -312.0566616799260373, 24.99999999999997158, 419.2731246273838792 ) ) ;
#4910=CARTESIAN_POINT ( 'NONE',  ( 11.81831109762787690, 2.222614453595284090E-15, 46.95220429669389262 ) ) ;
#4911=ORIENTED_EDGE ( 'NONE', *, *, #2524, .T. ) ;
#4912=CARTESIAN_POINT ( 'NONE',  ( -264.1404626571541598, 24.99999999999997158, 511.7445549721641100 ) ) ;
#4913=CIRCLE ( 'NONE', #4483, 1.000000000000000888 ) ;
#4915=CARTESIAN_POINT ( 'NONE',  ( -378.9271552156734515, 5.590393151250690779E-15, 174.6149733621406028 ) ) ;
#4919=FACE_OUTER_BOUND ( 'NONE', #425, .T. ) ;
#4920=FACE_OUTER_BOUND ( 'NONE', #3573, .T. ) ;
#4922=CARTESIAN_POINT ( 'NONE',  ( -353.5191290882918338, 0.000000000000000000, 198.1028895811323025 ) ) ;
#4923=DIRECTION ( 'NONE',  ( -0.9955873536034882676, 5.498835694391114214E-31, -0.09383933793885514130 ) ) ;
#4925=EDGE_CURVE ( 'NONE', #1574, #2554, #646, .T. ) ;
#4926=DIRECTION ( 'NONE',  ( 0.09383933793885568253, -2.673190762809473730E-31, -0.9955873536034882676 ) ) ;
#4927=MANIFOLD_SOLID_BREP ( 'Sweep1', #4461 ) ;
#4931=CARTESIAN_POINT ( 'NONE',  ( -353.4921497144319460, 2.222614453595284090E-15, 38.40071206960160310 ) ) ;
#4932=CARTESIAN_POINT ( 'NONE',  ( -360.7307227603793649, 2.222614453595284090E-15, 354.4373729494858480 ) ) ;
#4934=CIRCLE ( 'NONE', #2833, 23.00000000000121503 ) ;
#4936=AXIS2_PLACEMENT_3D ( 'NONE', #629, #2309, #3996 ) ;
#4938=AXIS2_PLACEMENT_3D ( 'NONE', #4873, #199, #2843 ) ;
#4939=CARTESIAN_POINT ( 'NONE',  ( -367.0460729392618191, 25.00000000000018474, 268.0688838304706678 ) ) ;
#4941=CARTESIAN_POINT ( 'NONE',  ( -207.8397519515728504, 5.421010862427522170E-17, 541.5412455041541762 ) ) ;
#4944=AXIS2_PLACEMENT_3D ( 'NONE', #1448, #3099, #4769 ) ;
#4946=CARTESIAN_POINT ( 'NONE',  ( 11.35554381052501682, 25.00000000000018474, 353.5846600851141943 ) ) ;
#4949=CARTESIAN_POINT ( 'NONE',  ( -351.7361816674535362, 5.421010862427522170E-17, 179.1867298626658283 ) ) ;
#4950=AXIS2_PLACEMENT_3D ( 'NONE', #4602, #2489, #1652 ) ;
#4951=AXIS2_PLACEMENT_3D ( 'NONE', #1970, #1141, #4494 ) ;
#4954=AXIS2_PLACEMENT_3D ( 'NONE', #3603, #268, #4100 ) ;
#4955=AXIS2_PLACEMENT_3D ( 'NONE', #2129, #1712, #5062 ) ;
#4956=ORIENTED_EDGE ( 'NONE', *, *, #2982, .T. ) ;
#4958=DIRECTION ( 'NONE',  ( 0.09383933793885537722, -2.626968444144180508E-31, -0.9955873536034883786 ) ) ;
#4959=DIRECTION ( 'NONE',  ( -1.219242865862094703E-16, 1.000000000000000000, -1.149200448409285278E-17 ) ) ;
#4962=ADVANCED_FACE ( 'NONE', ( #1594 ), #1352, .T. ) ;
#4966=CARTESIAN_POINT ( 'NONE',  ( -378.1800370315194186, 2.571758278209485443E-15, 235.9557576285559151 ) ) ;
#4967=ADVANCED_FACE ( 'NONE', ( #1645 ), #3788, .T. ) ;
#4971=CARTESIAN_POINT ( 'NONE',  ( 8.821273309659243722, 25.00000000000018474, 380.5076279642384520 ) ) ;
#4972=CARTESIAN_POINT ( 'NONE',  ( -223.9642223310802649, -25.00000000000003197, 534.3227077390027944 ) ) ;
#4976=CARTESIAN_POINT ( 'NONE',  ( -353.5191290882918338, 0.000000000000000000, 198.1028895811327573 ) ) ;
#4977=MANIFOLD_SOLID_BREP ( 'Boss-Extrude1', #3147 ) ;
#4982=DIRECTION ( 'NONE',  ( -1.219242865862094703E-16, 1.000000000000000000, -1.149200448409289593E-17 ) ) ;
#4983=CIRCLE ( 'NONE', #3242, 28.50000000000127898 ) ;
#4985=VERTEX_POINT ( 'NONE', #4571 ) ;
#4988=DIRECTION ( 'NONE',  ( -0.9955873536034882676, 5.452307672560250687E-31, -0.09383933793885569641 ) ) ;
#4989=CARTESIAN_POINT ( 'NONE',  ( -321.8445680969931004, 4.999156891862629509E-15, 103.6584595401686357 ) ) ;
#4990=CARTESIAN_POINT ( 'NONE',  ( -12.39202333278749357, 1.572093150103981429E-15, 98.84296066633379496 ) ) ;
#4991=CARTESIAN_POINT ( 'NONE',  ( -8.629236981521737349, 1.572093150103981429E-15, 142.6115645898827893 ) ) ;
#4992=DIRECTION ( 'NONE',  ( -0.9955873536034882676, 5.453577263127812432E-31, -0.09383933793885552987 ) ) ;
#4993=EDGE_CURVE ( 'NONE', #1199, #2087, #1261, .T. ) ;
#4996=CARTESIAN_POINT ( 'NONE',  ( -353.5191290882918338, 0.000000000000000000, 198.1028895811323025 ) ) ;
#4997=CARTESIAN_POINT ( 'NONE',  ( -353.5191290882918338, 0.000000000000000000, 198.1028895811327573 ) ) ;
#4998=ORIENTED_EDGE ( 'NONE', *, *, #1228, .T. ) ;
#5002=DIRECTION ( 'NONE',  ( -0.9955873536034882676, 5.452980219524763634E-31, -0.09383933793885573804 ) ) ;
#5003=DIRECTION ( 'NONE',  ( -0.9955873536034886007, 6.162975822039140717E-31, -0.09383933793885225472 ) ) ;
#5004=FACE_OUTER_BOUND ( 'NONE', #973, .T. ) ;
#5007=DIRECTION ( 'NONE',  ( -0.9955873536034882676, 5.452980219524763634E-31, -0.09383933793885573804 ) ) ;
#5009=DIRECTION ( 'NONE',  ( 0.09383933793885537722, -2.626968444144180508E-31, -0.9955873536034883786 ) ) ;
#5011=CARTESIAN_POINT ( 'NONE',  ( -152.2642418386349163, 3.740497495074990297E-15, 532.1805559224781064 ) ) ;
#5012=CARTESIAN_POINT ( 'NONE',  ( 11.65205807320734976, 3.740497495074990297E-15, 340.0738060255405912 ) ) ;
#5014=AXIS2_PLACEMENT_3D ( 'NONE', #2319, #668, #4898 ) ;
#5016=ORIENTED_EDGE ( 'NONE', *, *, #1325, .F. ) ;
#5020=DIRECTION ( 'NONE',  ( -5.679099018122554920E-31, -1.000000000000000000, 2.149753974990777610E-31 ) ) ;
#5021=EDGE_CURVE ( 'NONE', #861, #4306, #35, .T. ) ;
#5025=AXIS2_PLACEMENT_3D ( 'NONE', #3588, #5246, #2721 ) ;
#5026=CIRCLE ( 'NONE', #302, 4.382543221487789076 ) ;
#5027=DIRECTION ( 'NONE',  ( -0.09383933793885568253, 2.673190762809473730E-31, 0.9955873536034882676 ) ) ;
#5028=CARTESIAN_POINT ( 'NONE',  ( -357.8553543223658835, 2.759321206427282701E-15, 37.98945711520877211 ) ) ;
#5032=AXIS2_PLACEMENT_3D ( 'NONE', #1965, #2346, #1575 ) ;
#5034=CIRCLE ( 'NONE', #4869, 31.50000000000120082 ) ;
#5037=VERTEX_POINT ( 'NONE', #416 ) ;
#5039=CIRCLE ( 'NONE', #1359, 1.000000000000000888 ) ;
#5041=CARTESIAN_POINT ( 'NONE',  ( -373.4844736152189171, 3.367778697655401957E-15, 116.8709068531373703 ) ) ;
#5042=CARTESIAN_POINT ( 'NONE',  ( 6.585909452853061730, 3.740497495074990297E-15, 393.9228865916071527 ) ) ;
#5043=CARTESIAN_POINT ( 'NONE',  ( -336.1069982926118769, 1.517883041479706208E-15, 349.6877309229317916 ) ) ;
#5048=CARTESIAN_POINT ( 'NONE',  ( -330.7350079038403123, 5.421010862426367228E-17, 180.1617686057784056 ) ) ;
#5050=VERTEX_POINT ( 'NONE', #1 ) ;
#5052=CARTESIAN_POINT ( 'NONE',  ( -338.5986743560152377, -14.95948628165117178, 39.80450035817695209 ) ) ;
#5058=ORIENTED_EDGE ( 'NONE', *, *, #1635, .F. ) ;
#5060=VERTEX_POINT ( 'NONE', #3362 ) ;
#5062=DIRECTION ( 'NONE',  ( -0.9955873536034881566, 5.462637660443544243E-31, -0.09383933793885600172 ) ) ;
#5070=CARTESIAN_POINT ( 'NONE',  ( -63.04765821499436385, 1.843143693225357538E-15, 521.0401840782876661 ) ) ;
#5077=CARTESIAN_POINT ( 'NONE',  ( -338.5986743560152377, 14.95948628165116823, 39.80450035817695209 ) ) ;
#5078=CARTESIAN_POINT ( 'NONE',  ( -107.0991749147297014, -24.99999999999981881, 535.0680222229608489 ) ) ;
#5079=( LENGTH_UNIT ( ) NAMED_UNIT ( * ) SI_UNIT ( .MILLI., .METRE. ) );
#5081=CARTESIAN_POINT ( 'NONE',  ( -0.6802310551622114954, 2.222614453595284090E-15, 47.14310755735262859 ) ) ;
#5086=ADVANCED_FACE ( 'NONE', ( #55, #2591 ), #1727, .T. ) ;
#5088=FACE_BOUND ( 'NONE', #2399, .T. ) ;
#5089=EDGE_CURVE ( 'NONE', #3674, #4331, #2375, .T. ) ;
#5091=PLANE ( 'NONE',  #4783 ) ;
#5092=ADVANCED_FACE ( 'NONE', ( #4919 ), #4053, .F. ) ;
#5095=CARTESIAN_POINT ( 'NONE',  ( -344.8278606858024204, 3.635192770030907673E-30, 239.0993754495075621 ) ) ;
#5096=CARTESIAN_POINT ( 'NONE',  ( -198.3455225866217404, 1.517883041479706208E-15, 518.3576047634792303 ) ) ;
#5099=TOROIDAL_SURFACE ( 'NONE', #102, 28.50000000000115463, 1.000000000000000000 ) ;
#5107=CARTESIAN_POINT ( 'NONE',  ( 36.66581985038869362, 3.252606517456513302E-16, 340.1662229844753256 ) ) ;
#5109=CARTESIAN_POINT ( 'NONE',  ( -315.6465677682754176, 5.957787190994864669E-15, 121.3180010999883791 ) ) ;
#5110=CARTESIAN_POINT ( 'NONE',  ( -312.0566616799260373, -25.00000000000003197, 419.2731246273838792 ) ) ;
#5112=VECTOR ( 'NONE', #4549, 1000.000000000000114 ) ;
#5116=ORIENTED_EDGE ( 'NONE', *, *, #4654, .T. ) ;
#5120=DIRECTION ( 'NONE',  ( -0.9955873536034883786, 5.497582812564159916E-31, -0.09383933793885515517 ) ) ;
#5121=CARTESIAN_POINT ( 'NONE',  ( -353.4921497144319460, 2.222614453595284090E-15, 38.40071206960160310 ) ) ;
#5122=AXIS2_PLACEMENT_3D ( 'NONE', #3123, #998, #943 ) ;
#5127=CIRCLE ( 'NONE', #1181, 22.67218956682437536 ) ;
#5128=CIRCLE ( 'NONE', #2762, 31.50000000000120082 ) ;
#5130=CARTESIAN_POINT ( 'NONE',  ( -14.89480152442229688, 0.000000000000000000, 508.6517828409968729 ) ) ;
#5131=( GEOMETRIC_REPRESENTATION_CONTEXT ( 3 ) GLOBAL_UNCERTAINTY_ASSIGNED_CONTEXT ( ( #5170 ) ) GLOBAL_UNIT_ASSIGNED_CONTEXT ( ( #5079, #3427, #1888 ) ) REPRESENTATION_CONTEXT ( 'NONE', 'WORKASPACE' ) );
#5134=EDGE_LOOP ( 'NONE', ( #198, #5146, #1721, #4305 ) ) ;
#5137=EDGE_LOOP ( 'NONE', ( #1048, #3132, #1275, #712 ) ) ;
#5138=CARTESIAN_POINT ( 'NONE',  ( -367.0882437885061904, 2.222614453595284090E-15, 297.8351940652699454 ) ) ;
#5139=ORIENTED_EDGE ( 'NONE', *, *, #1030, .T. ) ;
#5141=ADVANCED_FACE ( 'NONE', ( #5226 ), #1992, .F. ) ;
#5142=CARTESIAN_POINT ( 'NONE',  ( -63.04765821500757284, -24.99999999999981881, 521.0401840782880072 ) ) ;
#5146=ORIENTED_EDGE ( 'NONE', *, *, #2765, .T. ) ;
#5148=CARTESIAN_POINT ( 'NONE',  ( -0.6802310551622114954, 2.222614453595284090E-15, 47.14310755735262859 ) ) ;
#5149=DIRECTION ( 'NONE',  ( -0.9955873536034882676, 5.498529991225532086E-31, -0.09383933793885536334 ) ) ;
#5150=DIRECTION ( 'NONE',  ( 0.9955873536034882676, -5.273458392682099492E-31, 0.09383933793885600172 ) ) ;
#5151=AXIS2_PLACEMENT_3D ( 'NONE', #4931, #647, #1913 ) ;
#5154=DIRECTION ( 'NONE',  ( -5.720779902258401340E-31, -1.000000000000000000, 2.099398147291833041E-31 ) ) ;
#5155=CARTESIAN_POINT ( 'NONE',  ( 24.85474708473260108, -25.00000000000000355, 216.1905617304888665 ) ) ;
#5157=CIRCLE ( 'NONE', #1383, 22.67218956682437536 ) ;
#5159=ORIENTED_EDGE ( 'NONE', *, *, #2208, .F. ) ;
#5160=CARTESIAN_POINT ( 'NONE',  ( -122.4270646331731598, 3.252606517456513302E-16, 560.5113017241549187 ) ) ;
#5163=ORIENTED_EDGE ( 'NONE', *, *, #894, .F. ) ;
#5164=CARTESIAN_POINT ( 'NONE',  ( -72.60637664584184847, 3.252606517456513302E-16, 552.9197695054128872 ) ) ;
#5165=ORIENTED_EDGE ( 'NONE', *, *, #2496, .F. ) ;
#5170=UNCERTAINTY_MEASURE_WITH_UNIT (LENGTH_MEASURE( 1.000000000000000082E-05 ), #5079, 'distance_accuracy_value', 'NONE');
#5175=EDGE_CURVE ( 'NONE', #4078, #3769, #3213, .T. ) ;
#5178=DIRECTION ( 'NONE',  ( 0.09383933793885537722, -2.626968444144180508E-31, -0.9955873536034883786 ) ) ;
#5179=CARTESIAN_POINT ( 'NONE',  ( -207.8397519515722252, -25.00000000000003197, 541.5412455041529256 ) ) ;
#5182=CARTESIAN_POINT ( 'NONE',  ( -360.7307227603793649, 2.222614453595284090E-15, 354.4373729494858480 ) ) ;
#5186=CARTESIAN_POINT ( 'NONE',  ( -30.63277980166709114, 25.00000000000018474, 527.1358351633700750 ) ) ;
#5188=EDGE_CURVE ( 'NONE', #4435, #3915, #635, .T. ) ;
#5190=DIRECTION ( 'NONE',  ( -0.9955873536034882676, 5.502656983963203831E-31, -0.09383933793885550212 ) ) ;
#5191=PLANE ( 'NONE',  #5122 ) ;
#5192=AXIS2_PLACEMENT_3D ( 'NONE', #5313, #2405, #752 ) ;
#5194=CIRCLE ( 'NONE', #5282, 21.00000000000124700 ) ;
#5196=EDGE_LOOP ( 'NONE', ( #2097, #1750 ) ) ;
#5198=DIRECTION ( 'NONE',  ( -0.09383933793885568253, 2.673190762809473730E-31, 0.9955873536034882676 ) ) ;
#5201=VECTOR ( 'NONE', #1367, 1000.000000000000114 ) ;
#5206=CARTESIAN_POINT ( 'NONE',  ( -345.9181427152443007, 2.222614453595284090E-15, 117.4603139392499429 ) ) ;
#5207=AXIS2_PLACEMENT_3D ( 'NONE', #696, #589, #2379 ) ;
#5208=CARTESIAN_POINT ( 'NONE',  ( -105.2090356704102447, -24.99999999999981881, 560.1816718768288865 ) ) ;
#5212=TOROIDAL_SURFACE ( 'NONE', #1533, 30.50000000000105516, 1.000000000000000000 ) ;
#5214=CARTESIAN_POINT ( 'NONE',  ( -105.2090356704105147, 2.222614453595284090E-15, 560.1816718768288865 ) ) ;
#5218=CARTESIAN_POINT ( 'NONE',  ( 24.85474708473287109, 3.252606517456513302E-16, 216.1905617304896623 ) ) ;
#5223=ORIENTED_EDGE ( 'NONE', *, *, #3615, .T. ) ;
#5226=FACE_OUTER_BOUND ( 'NONE', #1328, .T. ) ;
#5229=CARTESIAN_POINT ( 'NONE',  ( -330.6206199554102341, 2.816687638039051980E-15, 200.2611943537262107 ) ) ;
#5233=FACE_OUTER_BOUND ( 'NONE', #4358, .T. ) ;
#5234=CARTESIAN_POINT ( 'NONE',  ( 16.26935751051944479, 3.252606517456513302E-16, 140.3055424402290896 ) ) ;
#5237=DIRECTION ( 'NONE',  ( -0.09383933793885568253, 2.673190762809473730E-31, 0.9955873536034882676 ) ) ;
#5238=CARTESIAN_POINT ( 'NONE',  ( 18.31346110193259946, 25.00000000000018474, 444.2932575970297648 ) ) ;
#5240=CARTESIAN_POINT ( 'NONE',  ( 34.60640066538617532, -24.99999999999981881, 295.6817845355782879 ) ) ;
#5241=AXIS2_PLACEMENT_3D ( 'NONE', #2738, #4421, #2330 ) ;
#5242=EDGE_LOOP ( 'NONE', ( #3244, #98, #2189, #4901 ) ) ;
#5243=CARTESIAN_POINT ( 'NONE',  ( 6.585909452853061730, 3.740497495074990297E-15, 393.9228865916071527 ) ) ;
#5244=VERTEX_POINT ( 'NONE', #1931 ) ;
#5246=DIRECTION ( 'NONE',  ( -1.219242865862094703E-16, 1.000000000000000000, -1.149200448409289593E-17 ) ) ;
#5248=ORIENTED_EDGE ( 'NONE', *, *, #5308, .F. ) ;
#5253=ADVANCED_FACE ( 'NONE', ( #4813 ), #1162, .T. ) ;
#5256=EDGE_CURVE ( 'NONE', #2877, #281, #4417, .T. ) ;
#5258=CARTESIAN_POINT ( 'NONE',  ( -344.1351952944061168, 5.421010862427522170E-17, 98.54415422078321285 ) ) ;
#5261=DIRECTION ( 'NONE',  ( -0.9955873536034883786, 5.497582812564159916E-31, -0.09383933793885515517 ) ) ;
#5262=DIRECTION ( 'NONE',  ( -0.9955873536034881566, 5.462637660443544243E-31, -0.09383933793885600172 ) ) ;
#5264=CARTESIAN_POINT ( 'NONE',  ( -223.9642223310785312, 5.421010862427522170E-17, 534.3227077389987016 ) ) ;
#5265=CARTESIAN_POINT ( 'NONE',  ( -213.0979982360503584, 1.517883041479706208E-15, 511.7519955242227070 ) ) ;
#5266=CARTESIAN_POINT ( 'NONE',  ( -377.1442077948352107, 5.590393151250686046E-15, 155.6988136436743559 ) ) ;
#5268=CARTESIAN_POINT ( 'NONE',  ( -35.15684241565268309, 25.00000000000018474, 493.9702760599490716 ) ) ;
#5270=DIRECTION ( 'NONE',  ( -0.01527226085271972227, -2.080004339938201146E-31, -0.9998833722232041143 ) ) ;
#5271=EDGE_CURVE ( 'NONE', #3541, #3680, #818, .T. ) ;
#5272=VECTOR ( 'NONE', #3863, 1000.000000000000000 ) ;
#5274=ORIENTED_EDGE ( 'NONE', *, *, #1471, .F. ) ;
#5278=DIRECTION ( 'NONE',  ( -0.09383933793885568253, 2.673190762809473730E-31, 0.9955873536034882676 ) ) ;
#5281=VERTEX_POINT ( 'NONE', #4599 ) ;
#5282=AXIS2_PLACEMENT_3D ( 'NONE', #253, #1872, #5190 ) ;
#5285=DIRECTION ( 'NONE',  ( 0.09383933793885537722, -2.626968444144180508E-31, -0.9955873536034883786 ) ) ;
#5286=FACE_OUTER_BOUND ( 'NONE', #1106, .T. ) ;
#5287=CARTESIAN_POINT ( 'NONE',  ( -0.8482259245422840710, 2.276824562219559311E-15, 36.14439046289818691 ) ) ;
#5291=CIRCLE ( 'NONE', #1790, 28.50000000000127898 ) ;
#5294=CARTESIAN_POINT ( 'NONE',  ( -320.6447527397745034, 24.99999999999997158, 453.8399743637903612 ) ) ;
#5295=CARTESIAN_POINT ( 'NONE',  ( 36.66581985038869362, 3.252606517456513302E-16, 340.1662229844753256 ) ) ;
#5299=CIRCLE ( 'NONE', #4261, 17.00000000000009948 ) ;
#5301=CARTESIAN_POINT ( 'NONE',  ( -336.1069982926114221, 25.00000000000018474, 349.6877309229307684 ) ) ;
#5303=EDGE_LOOP ( 'NONE', ( #1801, #3967, #2994, #938 ) ) ;
#5308=EDGE_CURVE ( 'NONE', #3702, #744, #836, .T. ) ;
#5309=( GEOMETRIC_REPRESENTATION_CONTEXT ( 3 ) GLOBAL_UNCERTAINTY_ASSIGNED_CONTEXT ( ( #4895 ) ) GLOBAL_UNIT_ASSIGNED_CONTEXT ( ( #1289, #3033, #4348 ) ) REPRESENTATION_CONTEXT ( 'NONE', 'WORKASPACE' ) );
#5313=CARTESIAN_POINT ( 'NONE',  ( -353.4252897503525332, 0.000000000000000000, 197.1073022275279243 ) ) ;
#5316=EDGE_LOOP ( 'NONE', ( #1075, #120, #3118, #2621 ) ) ;
#5318=DIRECTION ( 'NONE',  ( 0.9955873536034882676, -5.498835694391114214E-31, 0.09383933793885514130 ) ) ;
#5319=DIRECTION ( 'NONE',  ( -0.09383933793885568253, 2.673190762809473730E-31, 0.9955873536034882676 ) ) ;
#5320=CARTESIAN_POINT ( 'NONE',  ( -351.5485029915759583, 2.222614453595284090E-15, 177.1955551554592603 ) ) ;
#5323=CARTESIAN_POINT ( 'NONE',  ( -167.9289969670495282, 25.00000000000018474, 528.5729890193230176 ) ) ;
#5324=CARTESIAN_POINT ( 'NONE',  ( -14.89480152442229688, 0.000000000000000000, 508.6517828409968729 ) ) ;
#5325=ORIENTED_EDGE ( 'NONE', *, *, #1206, .T. ) ;
#5326=CARTESIAN_POINT ( 'NONE',  ( -12.39202333278750601, 25.00000000000000355, 98.84296066633362443 ) ) ;
#5327=ORIENTED_EDGE ( 'NONE', *, *, #1221, .F. ) ;
#5329=TOROIDAL_SURFACE ( 'NONE', #1294, 30.50000000000105516, 1.000000000000000000 ) ;
#5331=VECTOR ( 'NONE', #136, 1000.000000000000114 ) ;
#5332=CARTESIAN_POINT ( 'NONE',  ( -346.0119820531829191, 0.000000000000000000, 118.4559012928527721 ) ) ;
#5335=AXIS2_PLACEMENT_3D ( 'NONE', #1528, #2795, #4560 ) ;
#5338=ORIENTED_EDGE ( 'NONE', *, *, #4380, .F. ) ;
#5340=DIRECTION ( 'NONE',  ( -0.09383933793885537722, 2.626968444144180508E-31, 0.9955873536034883786 ) ) ;
#5342=LINE ( 'NONE', #4055, #2043 ) ;
#5343=CARTESIAN_POINT ( 'NONE',  ( -357.2727026058461206, 5.421010862427522170E-17, 237.9263837252718758 ) ) ;
#5345=EDGE_LOOP ( 'NONE', ( #2467, #3482 ) ) ;
#5352=CARTESIAN_POINT ( 'NONE',  ( -156.9923520473274721, 25.00000000000018474, 556.8176423728723421 ) ) ;
#5353=CARTESIAN_POINT ( 'NONE',  ( 29.77542608467492613, 2.222614453595284090E-15, 249.2409987768030533 ) ) ;
#5355=CARTESIAN_POINT ( 'NONE',  ( -48.20943979671786650, 25.00000000000018474, 509.2978244404892507 ) ) ;
#5356=ORIENTED_EDGE ( 'NONE', *, *, #2341, .T. ) ;
#5357=DIRECTION ( 'NONE',  ( 0.09383933793885568253, -2.673190762809473730E-31, -0.9955873536034882676 ) ) ;
#5358=EDGE_CURVE ( 'NONE', #251, #1398, #1239, .T. ) ;
#5361=ADVANCED_FACE ( 'NONE', ( #2461 ), #4163, .F. ) ;
#5362=ORIENTED_EDGE ( 'NONE', *, *, #111, .T. ) ;
#5363=CARTESIAN_POINT ( 'NONE',  ( -338.5986743560152377, -14.95948628165117178, 39.80450035817695209 ) ) ;
#5364=CARTESIAN_POINT ( 'NONE',  ( -323.0598754654449181, 3.735172737399573480E-15, 199.9694020346631191 ) ) ;
#5366=CARTESIAN_POINT ( 'NONE',  ( -369.7175445258896502, 1.530808498934214793E-15, 236.7533920010361896 ) ) ;
#5369=AXIS2_PLACEMENT_3D ( 'NONE', #149, #4384, #2246 ) ;
#5370=ORIENTED_EDGE ( 'NONE', *, *, #2816, .T. ) ;
#5373=CARTESIAN_POINT ( 'NONE',  ( -321.8445680969931004, 4.999156891862629509E-15, 103.6584595401686215 ) ) ;
#5375=DIRECTION ( 'NONE',  ( -0.09383933793885537722, 2.626968444144180508E-31, 0.9955873536034883786 ) ) ;
#5376=AXIS2_PLACEMENT_3D ( 'NONE', #5077, #1703, #1321 ) ;
#5379=CARTESIAN_POINT ( 'NONE',  ( 0.07030049710132768581, 1.843143693225357538E-15, 219.5055207296747710 ) ) ;
#5381=CARTESIAN_POINT ( 'NONE',  ( -320.6447527397726276, 2.276824562219559311E-15, 453.8399743637901906 ) ) ;
#5382=AXIS2_PLACEMENT_3D ( 'NONE', #2960, #3050, #4227 ) ;
#5383=EDGE_LOOP ( 'NONE', ( #3921, #2215, #1828, #3177 ) ) ;
#5384=ORIENTED_EDGE ( 'NONE', *, *, #4460, .T. ) ;
#5387=( NAMED_UNIT ( * ) PLANE_ANGLE_UNIT ( ) SI_UNIT ( $, .RADIAN. ) );
#5390=AXIS2_PLACEMENT_3D ( 'NONE', #1768, #2653, #562 ) ;
#5391=PRODUCT_DEFINITION_SHAPE ( 'NONE', 'NONE',  #3211 ) ;
#5393=CARTESIAN_POINT ( 'NONE',  ( -323.7051989975983588, 2.222614453595284090E-15, 41.20828864675230108 ) ) ;
#5399=CIRCLE ( 'NONE', #3043, 17.00000000000009948 ) ;
#5401=LINE ( 'NONE', #4636, #2238 ) ;
#5403=CARTESIAN_POINT ( 'NONE',  ( -319.3419943896644213, 2.222614453595281723E-15, 41.61954360114513207 ) ) ;
#5405=CARTESIAN_POINT ( 'NONE',  ( -52.92425795464261995, 3.794707603699265519E-15, 513.6488213284153517 ) ) ;
#5406=CARTESIAN_POINT ( 'NONE',  ( -367.0882437885064746, 25.00000000000018474, 297.8351940652706276 ) ) ;
#5407=CARTESIAN_POINT ( 'NONE',  ( -49.96441683051492078, -24.99999999999981881, 542.4422122871054626 ) ) ;
#5418=FACE_BOUND ( 'NONE', #3944, .T. ) ;
#5419=CLOSED_SHELL ( 'NONE', ( #4583, #2308, #3847, #4761, #1597, #402 ) ) ;
#5420=ORIENTED_EDGE ( 'NONE', *, *, #1917, .T. ) ;
#5422=DIRECTION ( 'NONE',  ( -1.000000000000000000, -1.219242865862094703E-16, 0.000000000000000000 ) ) ;
#5423=CARTESIAN_POINT ( 'NONE',  ( -349.7655555707380017, 2.222614453595284090E-15, 158.2793954369929850 ) ) ;
#5424=DIRECTION ( 'NONE',  ( -0.09383933793885536334, 2.626968444144180070E-31, 0.9955873536034882676 ) ) ;
#5425=EDGE_CURVE ( 'NONE', #2290, #5037, #1427, .T. ) ;
#5427=DIRECTION ( 'NONE',  ( 0.09383933793885568253, -2.673190762809473730E-31, -0.9955873536034882676 ) ) ;
#5429=AXIS2_PLACEMENT_3D ( 'NONE', #778, #2896, #3294 ) ;
#5431=CARTESIAN_POINT ( 'NONE',  ( 10.82492224058167984, 3.740497495074990297E-15, 312.2165827548582229 ) ) ;
#5445=COLOUR_RGB('Light Blue',0.38,0.62,0.78);
#5446=FILL_AREA_STYLE_COLOUR('',#5445);
#5447=FILL_AREA_STYLE('',(#5446));
#5448=SURFACE_STYLE_FILL_AREA(#5447);
#5449=SURFACE_SIDE_STYLE('',(#5448));
#5450=SURFACE_STYLE_USAGE(.BOTH.,#5449);
#5451=PRESENTATION_STYLE_ASSIGNMENT((#5450));
ENDSEC;
END-ISO-10303-21;
